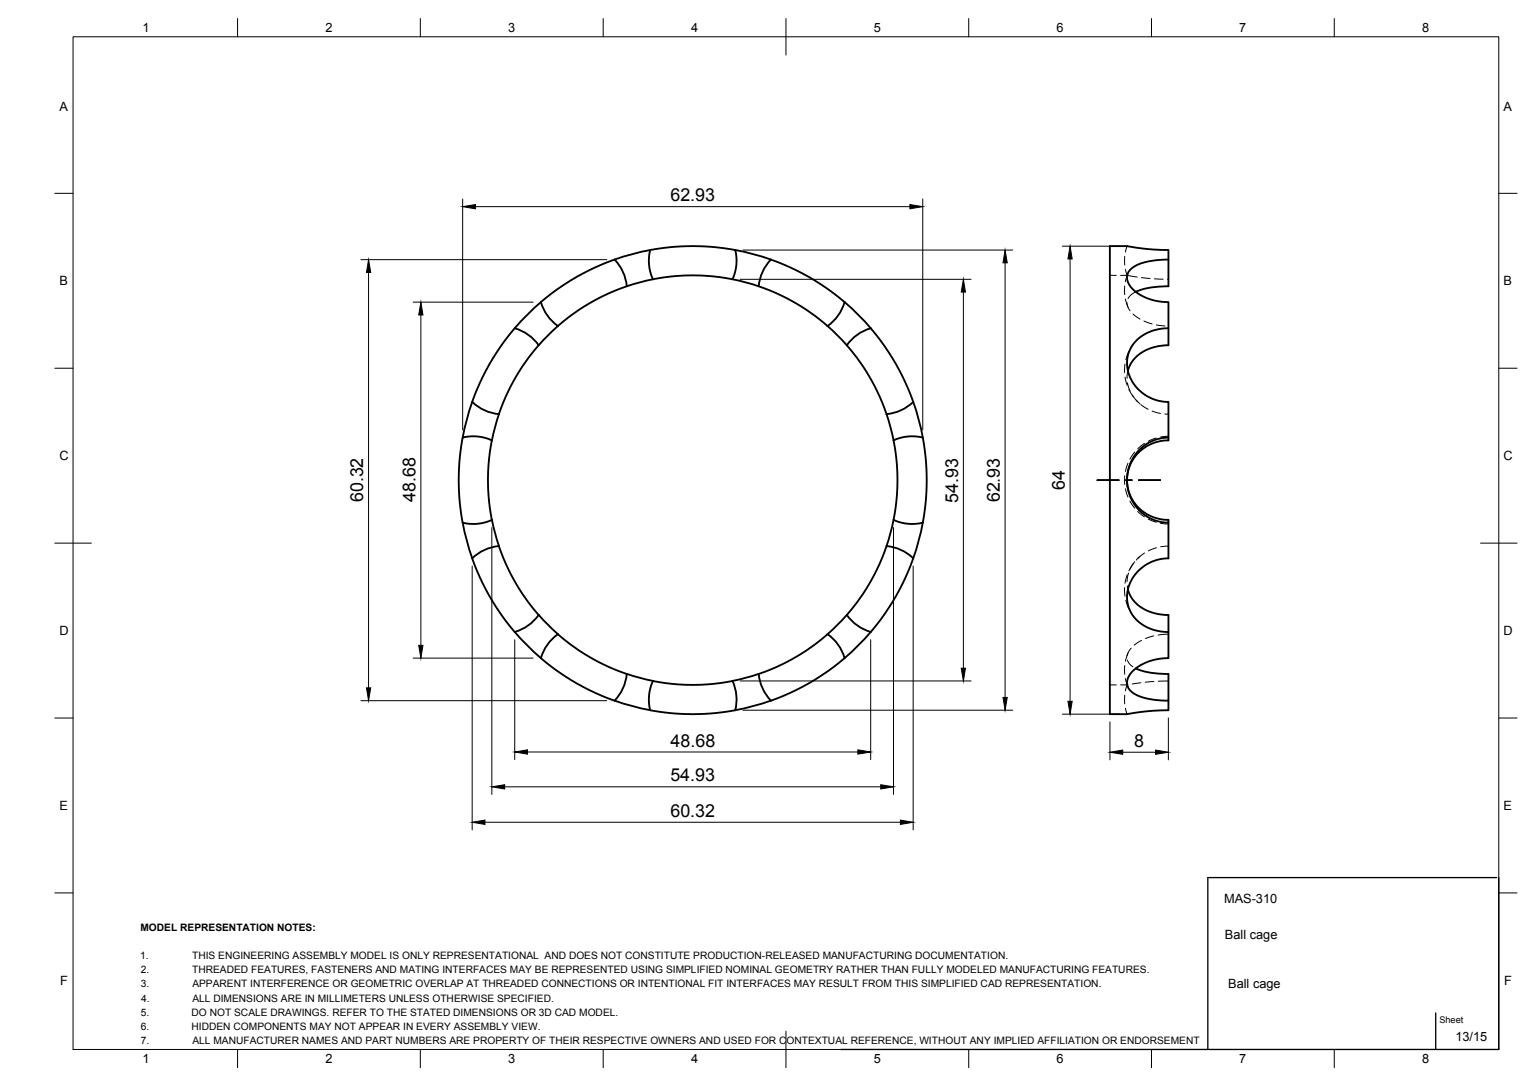
ISO-10303-21;
HEADER;
/* Generated by software containing ST-Developer
 * from STEP Tools, Inc. (www.steptools.com) 
 */

FILE_DESCRIPTION(
/* description */ ('Independent30mm screw-fed quill/spindle unit with16mm straight tool s
ocket, radial set screw, native reusable open ball bearings, retained 
inner/outer race stacks, keyed quill guide and M12x1.75 fine feed. Ext
ernal moving drive and tool not included. Ideal cage orbital links; in
dividual ball spin, force and preload not simulated. No drilling capac
ity, runout, speed, torque, load, life or machine safety rating.'),
/* implementation_level */ '2;1');

FILE_NAME(
/* name */ 'Ball cage.step',
/* time_stamp */ '2026-11-08T18:59:42-08:00',
/* author */ (''),
/* organization */ (''),
/* preprocessor_version */ 'ST-DEVELOPER v20.2',
/* originating_system */ 'Autodesk Translation Framework v15.17.0.0',
/* authorisation */ '');

FILE_SCHEMA (('AUTOMOTIVE_DESIGN { 1 0 10303 214 3 1 1 }'));
ENDSEC;

DATA;
#10=MECHANICAL_DESIGN_GEOMETRIC_PRESENTATION_REPRESENTATION('',(#1607),#63898);
#224=SPHERICAL_SURFACE('',#16652,6.);
#225=SPHERICAL_SURFACE('',#16673,6.);
#226=SPHERICAL_SURFACE('',#16679,6.);
#227=SPHERICAL_SURFACE('',#16686,6.);
#228=SPHERICAL_SURFACE('',#16692,6.);
#229=SPHERICAL_SURFACE('',#16698,6.);
#230=SPHERICAL_SURFACE('',#16704,6.);
#231=SPHERICAL_SURFACE('',#16710,6.);
#232=SPHERICAL_SURFACE('',#16717,6.);
#233=SPHERICAL_SURFACE('',#16723,6.);
#234=SPHERICAL_SURFACE('',#16729,6.);
#235=SPHERICAL_SURFACE('',#16735,6.);
#1448=B_SPLINE_CURVE_WITH_KNOTS('',3,(#60434,#60435,#60436,#60437,#60438,
#60439,#60440,#60441,#60442,#60443,#60444,#60445,#60446,#60447,#60448,#60449,
#60450,#60451,#60452,#60453,#60454,#60455,#60456,#60457,#60458,#60459),
 .UNSPECIFIED.,.F.,.F.,(4,2,2,2,2,2,2,2,2,2,2,2,4),(-1.71701449155744,-1.52195735713249,
-1.32690022270754,-1.23846982832783,-1.15003943394813,-1.00427333986342,
-0.858507245778717,-0.712741151694014,-0.56697505760931,-0.478544663229604,
-0.390114268849898,-0.195057134424949,0.),.UNSPECIFIED.);
#1449=B_SPLINE_CURVE_WITH_KNOTS('',3,(#60463,#60464,#60465,#60466,#60467,
#60468,#60469,#60470,#60471,#60472,#60473,#60474),.UNSPECIFIED.,.F.,.F.,
(4,2,2,2,2,4),(-0.73325034842368,-0.710785333485644,-0.57603622531241,-0.432027168984308,
-0.288018112656205,0.),.UNSPECIFIED.);
#1450=B_SPLINE_CURVE_WITH_KNOTS('',3,(#60478,#60479,#60480,#60481,#60482,
#60483,#60484,#60485,#60486,#60487,#60488,#60489,#60490,#60491),
 .UNSPECIFIED.,.F.,.F.,(4,2,2,2,2,2,4),(-1.69106888331775,-1.40305077066155,
-1.25904171433345,-1.11503265800535,-0.980283549832111,-0.845534441658878,
-0.73325034842368),.UNSPECIFIED.);
#1451=B_SPLINE_CURVE_WITH_KNOTS('',3,(#60499,#60500,#60501,#60502,#60503,
#60504,#60505,#60506,#60507,#60508,#60509,#60510),.UNSPECIFIED.,.F.,.F.,
(4,2,2,2,2,4),(-0.845534441658877,-0.710785333485644,-0.576036225312411,
-0.432027168984308,-0.288018112656205,0.),.UNSPECIFIED.);
#1452=B_SPLINE_CURVE_WITH_KNOTS('',3,(#60514,#60515,#60516,#60517,#60518,
#60519,#60520,#60521,#60522,#60523,#60524,#60525,#60526,#60527,#60528,#60529,
#60530,#60531,#60532,#60533,#60534,#60535),.UNSPECIFIED.,.F.,.F.,(4,2,2,
2,2,2,2,2,2,2,4),(-1.69106888331776,-1.40305077066155,-1.25904171433345,
-1.11503265800535,-0.980283549832111,-0.845534441658878,-0.710785333485644,
-0.57603622531241,-0.432027168984307,-0.288018112656205,0.),
 .UNSPECIFIED.);
#1453=B_SPLINE_CURVE_WITH_KNOTS('',3,(#60539,#60540,#60541,#60542,#60543,
#60544,#60545,#60546,#60547,#60548,#60549,#60550,#60551,#60552,#60553,#60554,
#60555,#60556,#60557,#60558,#60559,#60560),.UNSPECIFIED.,.F.,.F.,(4,2,2,
2,2,2,2,2,2,2,4),(-1.69106888331776,-1.40305077066155,-1.25904171433345,
-1.11503265800535,-0.980283549832111,-0.845534441658878,-0.710785333485644,
-0.57603622531241,-0.432027168984307,-0.288018112656205,0.),
 .UNSPECIFIED.);
#1454=B_SPLINE_CURVE_WITH_KNOTS('',3,(#60564,#60565,#60566,#60567,#60568,
#60569,#60570,#60571,#60572,#60573,#60574,#60575,#60576,#60577,#60578,#60579,
#60580,#60581,#60582,#60583,#60584,#60585),.UNSPECIFIED.,.F.,.F.,(4,2,2,
2,2,2,2,2,2,2,4),(-1.69106888331775,-1.40305077066155,-1.25904171433345,
-1.11503265800534,-0.980283549832111,-0.845534441658877,-0.710785333485644,
-0.57603622531241,-0.432027168984307,-0.288018112656205,0.),
 .UNSPECIFIED.);
#1455=B_SPLINE_CURVE_WITH_KNOTS('',3,(#60589,#60590,#60591,#60592,#60593,
#60594),.UNSPECIFIED.,.F.,.F.,(4,2,4),(-1.69106888331776,-1.40305077066155,
-1.27424252614337),.UNSPECIFIED.);
#1456=B_SPLINE_CURVE_WITH_KNOTS('',3,(#60596,#60597,#60598,#60599,#60600,
#60601,#60602,#60603,#60604,#60605,#60606,#60607,#60608,#60609,#60610,#60611,
#60612,#60613,#60614,#60615),.UNSPECIFIED.,.F.,.F.,(4,2,2,2,2,2,2,2,2,4),
(-1.27424252614337,-1.25904171433345,-1.11503265800534,-0.980283549832111,
-0.845534441658877,-0.710785333485643,-0.576036225312409,-0.432027168984307,
-0.288018112656205,0.),.UNSPECIFIED.);
#1457=B_SPLINE_CURVE_WITH_KNOTS('',3,(#60619,#60620,#60621,#60622,#60623,
#60624,#60625,#60626,#60627,#60628,#60629,#60630),.UNSPECIFIED.,.F.,.F.,
(4,2,2,2,2,4),(-1.69106888331776,-1.40305077066155,-1.25904171433345,-1.11503265800534,
-0.980283549832111,-0.957818534894075),.UNSPECIFIED.);
#1458=B_SPLINE_CURVE_WITH_KNOTS('',3,(#60632,#60633,#60634,#60635,#60636,
#60637,#60638,#60639,#60640,#60641,#60642,#60643,#60644,#60645),
 .UNSPECIFIED.,.F.,.F.,(4,2,2,2,2,2,4),(-0.957818534894075,-0.845534441658877,
-0.710785333485644,-0.57603622531241,-0.432027168984307,-0.288018112656205,
0.),.UNSPECIFIED.);
#1459=B_SPLINE_CURVE_WITH_KNOTS('',3,(#60649,#60650,#60651,#60652,#60653,
#60654,#60655,#60656,#60657,#60658,#60659,#60660),.UNSPECIFIED.,.F.,.F.,
(4,2,2,2,2,4),(-1.69106888331776,-1.40305077066155,-1.25904171433345,-1.11503265800535,
-0.980283549832111,-0.845534441658878),.UNSPECIFIED.);
#1460=B_SPLINE_CURVE_WITH_KNOTS('',3,(#60662,#60663,#60664,#60665,#60666,
#60667,#60668,#60669,#60670,#60671,#60672,#60673),.UNSPECIFIED.,.F.,.F.,
(4,2,2,2,2,4),(-0.845534441658878,-0.710785333485644,-0.57603622531241,
-0.432027168984308,-0.288018112656205,0.),.UNSPECIFIED.);
#1461=B_SPLINE_CURVE_WITH_KNOTS('',3,(#60678,#60679,#60680,#60681,#60682,
#60683,#60684,#60685,#60686,#60687,#60688,#60689,#60690,#60691,#60692,#60693,
#60694,#60695,#60696,#60697),.UNSPECIFIED.,.F.,.F.,(4,2,2,2,2,2,2,2,2,4),
(-1.69106888331775,-1.40305077066155,-1.25904171433345,-1.11503265800535,
-0.980283549832112,-0.845534441658878,-0.710785333485644,-0.57603622531241,
-0.432027168984308,-0.416826357174388),.UNSPECIFIED.);
#1462=B_SPLINE_CURVE_WITH_KNOTS('',3,(#60699,#60700,#60701,#60702,#60703,
#60704),.UNSPECIFIED.,.F.,.F.,(4,2,4),(-0.416826357174388,-0.288018112656205,
0.),.UNSPECIFIED.);
#1463=B_SPLINE_CURVE_WITH_KNOTS('',3,(#60708,#60709,#60710,#60711,#60712,
#60713,#60714,#60715,#60716,#60717,#60718,#60719,#60720,#60721,#60722,#60723,
#60724,#60725,#60726,#60727,#60728,#60729),.UNSPECIFIED.,.F.,.F.,(4,2,2,
2,2,2,2,2,2,2,4),(-1.69106888331776,-1.40305077066155,-1.25904171433345,
-1.11503265800535,-0.980283549832111,-0.845534441658878,-0.710785333485644,
-0.576036225312411,-0.432027168984308,-0.288018112656205,0.),
 .UNSPECIFIED.);
#1464=B_SPLINE_CURVE_WITH_KNOTS('',3,(#60733,#60734,#60735,#60736,#60737,
#60738,#60739,#60740,#60741,#60742,#60743,#60744,#60745,#60746,#60747,#60748,
#60749,#60750,#60751,#60752,#60753,#60754),.UNSPECIFIED.,.F.,.F.,(4,2,2,
2,2,2,2,2,2,2,4),(-1.69106888331776,-1.40305077066155,-1.25904171433345,
-1.11503265800535,-0.980283549832111,-0.845534441658878,-0.710785333485644,
-0.57603622531241,-0.432027168984308,-0.288018112656205,0.),
 .UNSPECIFIED.);
#1465=B_SPLINE_CURVE_WITH_KNOTS('',3,(#60758,#60759,#60760,#60761,#60762,
#60763,#60764,#60765,#60766,#60767,#60768,#60769,#60770,#60771,#60772,#60773,
#60774,#60775,#60776,#60777,#60778,#60779),.UNSPECIFIED.,.F.,.F.,(4,2,2,
2,2,2,2,2,2,2,4),(-1.69106888331776,-1.40305077066155,-1.25904171433345,
-1.11503265800535,-0.980283549832113,-0.845534441658879,-0.710785333485645,
-0.576036225312412,-0.432027168984308,-0.288018112656206,0.),
 .UNSPECIFIED.);
#1466=B_SPLINE_CURVE_WITH_KNOTS('',3,(#60782,#60783,#60784,#60785,#60786,
#60787,#60788,#60789,#60790,#60791,#60792,#60793),.UNSPECIFIED.,.F.,.F.,
(4,2,2,2,2,4),(-1.69106888331776,-1.40305077066155,-1.25904171433345,-1.11503265800535,
-0.980283549832112,-0.845534441658877),.UNSPECIFIED.);
#1467=B_SPLINE_CURVE_WITH_KNOTS('',3,(#60800,#60801,#60802,#60803,#60804,
#60805,#60806,#60807,#60808,#60809,#60810,#60811,#60812,#60813,#60814,#60815,
#60816,#60817,#60818,#60819,#60820,#60821,#60822,#60823,#60824,#60825),
 .UNSPECIFIED.,.F.,.F.,(4,2,2,2,2,2,2,2,2,2,2,2,4),(-1.71701449155743,-1.52195735713249,
-1.32690022270754,-1.23846982832783,-1.15003943394812,-1.00427333986342,
-0.858507245778717,-0.712741151694013,-0.56697505760931,-0.478544663229604,
-0.390114268849898,-0.195057134424949,0.),.UNSPECIFIED.);
#1468=B_SPLINE_CURVE_WITH_KNOTS('',3,(#60835,#60836,#60837,#60838,#60839,
#60840,#60841,#60842,#60843,#60844,#60845,#60846,#60847,#60848,#60849,#60850,
#60851,#60852,#60853,#60854,#60855,#60856,#60857,#60858,#60859,#60860),
 .UNSPECIFIED.,.F.,.F.,(4,2,2,2,2,2,2,2,2,2,2,2,4),(-1.71701449155744,-1.52195735713249,
-1.32690022270754,-1.23846982832783,-1.15003943394812,-1.00427333986342,
-0.858507245778718,-0.712741151694014,-0.56697505760931,-0.478544663229604,
-0.390114268849898,-0.195057134424949,0.),.UNSPECIFIED.);
#1469=B_SPLINE_CURVE_WITH_KNOTS('',3,(#60873,#60874,#60875,#60876,#60877,
#60878,#60879,#60880,#60881,#60882),.UNSPECIFIED.,.F.,.F.,(4,2,2,2,4),(-1.71701449155744,
-1.52195735713249,-1.32690022270754,-1.23846982832783,-1.17815521207059),
 .UNSPECIFIED.);
#1470=B_SPLINE_CURVE_WITH_KNOTS('',3,(#60884,#60885,#60886,#60887,#60888,
#60889,#60890,#60891,#60892,#60893,#60894,#60895,#60896,#60897,#60898,#60899,
#60900,#60901,#60902,#60903),.UNSPECIFIED.,.F.,.F.,(4,2,2,2,2,2,2,2,2,4),
(-1.17815521207059,-1.15003943394812,-1.00427333986342,-0.858507245778718,
-0.712741151694014,-0.56697505760931,-0.478544663229604,-0.390114268849898,
-0.195057134424949,0.),.UNSPECIFIED.);
#1471=B_SPLINE_CURVE_WITH_KNOTS('',3,(#60913,#60914,#60915,#60916,#60917,
#60918,#60919,#60920,#60921,#60922,#60923,#60924,#60925,#60926),
 .UNSPECIFIED.,.F.,.F.,(4,2,2,2,2,2,4),(-1.71701449155744,-1.52195735713249,
-1.32690022270754,-1.23846982832783,-1.15003943394813,-1.00427333986342,
-0.968278936736989),.UNSPECIFIED.);
#1472=B_SPLINE_CURVE_WITH_KNOTS('',3,(#60928,#60929,#60930,#60931,#60932,
#60933,#60934,#60935,#60936,#60937,#60938,#60939,#60940,#60941,#60942,#60943),
 .UNSPECIFIED.,.F.,.F.,(4,2,2,2,2,2,2,4),(-0.968278936736989,-0.858507245778719,
-0.712741151694015,-0.566975057609311,-0.478544663229605,-0.390114268849899,
-0.19505713442495,0.),.UNSPECIFIED.);
#1473=B_SPLINE_CURVE_WITH_KNOTS('',3,(#60953,#60954,#60955,#60956,#60957,
#60958,#60959,#60960,#60961,#60962,#60963,#60964,#60965,#60966),
 .UNSPECIFIED.,.F.,.F.,(4,2,2,2,2,2,4),(-1.71701449155743,-1.52195735713248,
-1.32690022270754,-1.23846982832783,-1.15003943394812,-1.00427333986342,
-0.858507245778716),.UNSPECIFIED.);
#1474=B_SPLINE_CURVE_WITH_KNOTS('',3,(#60968,#60969,#60970,#60971,#60972,
#60973,#60974,#60975,#60976,#60977,#60978,#60979,#60980,#60981),
 .UNSPECIFIED.,.F.,.F.,(4,2,2,2,2,2,4),(-0.858507245778716,-0.712741151694012,
-0.566975057609308,-0.478544663229602,-0.390114268849896,-0.195057134424948,
0.),.UNSPECIFIED.);
#1475=B_SPLINE_CURVE_WITH_KNOTS('',3,(#60991,#60992,#60993,#60994,#60995,
#60996,#60997,#60998,#60999,#61000,#61001,#61002,#61003,#61004,#61005,#61006),
 .UNSPECIFIED.,.F.,.F.,(4,2,2,2,2,2,2,4),(-1.71701449155744,-1.52195735713249,
-1.32690022270754,-1.23846982832783,-1.15003943394812,-1.00427333986342,
-0.858507245778716,-0.748735554820447),.UNSPECIFIED.);
#1476=B_SPLINE_CURVE_WITH_KNOTS('',3,(#61008,#61009,#61010,#61011,#61012,
#61013,#61014,#61015,#61016,#61017,#61018,#61019,#61020,#61021),
 .UNSPECIFIED.,.F.,.F.,(4,2,2,2,2,2,4),(-0.748735554820447,-0.712741151694013,
-0.56697505760931,-0.478544663229603,-0.390114268849895,-0.195057134424948,
0.),.UNSPECIFIED.);
#1477=B_SPLINE_CURVE_WITH_KNOTS('',3,(#61031,#61032,#61033,#61034,#61035,
#61036,#61037,#61038,#61039,#61040,#61041,#61042,#61043,#61044,#61045,#61046,
#61047,#61048,#61049,#61050),.UNSPECIFIED.,.F.,.F.,(4,2,2,2,2,2,2,2,2,4),
(-1.71701449155743,-1.52195735713249,-1.32690022270754,-1.23846982832783,
-1.15003943394812,-1.00427333986342,-0.858507245778717,-0.712741151694014,
-0.566975057609311,-0.538859279486847),.UNSPECIFIED.);
#1478=B_SPLINE_CURVE_WITH_KNOTS('',3,(#61052,#61053,#61054,#61055,#61056,
#61057,#61058,#61059,#61060,#61061),.UNSPECIFIED.,.F.,.F.,(4,2,2,2,4),(-0.538859279486847,
-0.478544663229605,-0.3901142688499,-0.19505713442495,0.),.UNSPECIFIED.);
#1479=B_SPLINE_CURVE_WITH_KNOTS('',3,(#61072,#61073,#61074,#61075,#61076,
#61077,#61078,#61079,#61080,#61081,#61082,#61083,#61084,#61085,#61086,#61087,
#61088,#61089,#61090,#61091,#61092,#61093,#61094,#61095,#61096,#61097),
 .UNSPECIFIED.,.F.,.F.,(4,2,2,2,2,2,2,2,2,2,2,2,4),(-1.71701449155743,-1.52195735713249,
-1.32690022270754,-1.23846982832783,-1.15003943394813,-1.00427333986342,
-0.858507245778717,-0.712741151694013,-0.56697505760931,-0.478544663229603,
-0.390114268849897,-0.195057134424949,0.),.UNSPECIFIED.);
#1480=B_SPLINE_CURVE_WITH_KNOTS('',3,(#61107,#61108,#61109,#61110,#61111,
#61112,#61113,#61114,#61115,#61116,#61117,#61118,#61119,#61120,#61121,#61122,
#61123,#61124,#61125,#61126,#61127,#61128,#61129,#61130,#61131,#61132),
 .UNSPECIFIED.,.F.,.F.,(4,2,2,2,2,2,2,2,2,2,2,2,4),(-1.71701449155743,-1.52195735713249,
-1.32690022270754,-1.23846982832783,-1.15003943394812,-1.00427333986342,
-0.858507245778718,-0.712741151694014,-0.56697505760931,-0.478544663229604,
-0.390114268849898,-0.195057134424949,0.),.UNSPECIFIED.);
#1481=B_SPLINE_CURVE_WITH_KNOTS('',3,(#61142,#61143,#61144,#61145,#61146,
#61147,#61148,#61149,#61150,#61151,#61152,#61153,#61154,#61155,#61156,#61157,
#61158,#61159,#61160,#61161,#61162,#61163,#61164,#61165,#61166,#61167),
 .UNSPECIFIED.,.F.,.F.,(4,2,2,2,2,2,2,2,2,2,2,2,4),(-1.71701449155744,-1.52195735713249,
-1.32690022270754,-1.23846982832783,-1.15003943394813,-1.00427333986342,
-0.858507245778718,-0.712741151694014,-0.56697505760931,-0.478544663229604,
-0.390114268849898,-0.195057134424949,0.),.UNSPECIFIED.);
#1482=B_SPLINE_CURVE_WITH_KNOTS('',3,(#61177,#61178,#61179,#61180,#61181,
#61182,#61183,#61184,#61185,#61186,#61187,#61188,#61189,#61190,#61191,#61192,
#61193,#61194,#61195,#61196,#61197,#61198,#61199,#61200,#61201,#61202),
 .UNSPECIFIED.,.F.,.F.,(4,2,2,2,2,2,2,2,2,2,2,2,4),(-1.71701449155743,-1.52195735713249,
-1.32690022270754,-1.23846982832783,-1.15003943394812,-1.00427333986342,
-0.858507245778717,-0.712741151694014,-0.56697505760931,-0.478544663229604,
-0.390114268849898,-0.195057134424949,0.),.UNSPECIFIED.);
#1571=SHAPE_REPRESENTATION_RELATIONSHIP('SRR','None',#64010,#1589);
#1589=ADVANCED_BREP_SHAPE_REPRESENTATION('',(#1625),#63895);
#1607=STYLED_ITEM('',(#64105),#1625);
#1625=MANIFOLD_SOLID_BREP('Body1',#15493);
#1710=FACE_BOUND('',#4365,.T.);
#2341=CYLINDRICAL_SURFACE('',#16656,28.);
#2342=CYLINDRICAL_SURFACE('',#16738,32.);
#2585=CIRCLE('',#16653,6.);
#2586=CIRCLE('',#16654,6.);
#2587=CIRCLE('',#16655,6.);
#2588=CIRCLE('',#16657,28.);
#2589=CIRCLE('',#16658,28.);
#2590=CIRCLE('',#16659,28.);
#2591=CIRCLE('',#16660,28.);
#2592=CIRCLE('',#16661,28.);
#2593=CIRCLE('',#16662,28.);
#2594=CIRCLE('',#16663,28.);
#2595=CIRCLE('',#16664,28.);
#2596=CIRCLE('',#16665,28.);
#2597=CIRCLE('',#16666,28.);
#2598=CIRCLE('',#16667,28.);
#2599=CIRCLE('',#16668,28.);
#2600=CIRCLE('',#16669,28.);
#2601=CIRCLE('',#16671,32.);
#2602=CIRCLE('',#16672,6.);
#2603=CIRCLE('',#16674,6.);
#2604=CIRCLE('',#16675,6.);
#2605=CIRCLE('',#16677,32.);
#2606=CIRCLE('',#16678,6.);
#2607=CIRCLE('',#16680,6.);
#2608=CIRCLE('',#16681,6.);
#2609=CIRCLE('',#16682,6.);
#2610=CIRCLE('',#16684,32.);
#2611=CIRCLE('',#16685,6.);
#2612=CIRCLE('',#16687,6.);
#2613=CIRCLE('',#16688,6.);
#2614=CIRCLE('',#16690,32.);
#2615=CIRCLE('',#16691,6.);
#2616=CIRCLE('',#16693,6.);
#2617=CIRCLE('',#16694,6.00000000000001);
#2618=CIRCLE('',#16696,32.);
#2619=CIRCLE('',#16697,6.);
#2620=CIRCLE('',#16699,6.);
#2621=CIRCLE('',#16700,6.);
#2622=CIRCLE('',#16702,32.);
#2623=CIRCLE('',#16703,6.);
#2624=CIRCLE('',#16705,6.);
#2625=CIRCLE('',#16706,6.);
#2626=CIRCLE('',#16708,32.);
#2627=CIRCLE('',#16709,6.);
#2628=CIRCLE('',#16711,6.);
#2629=CIRCLE('',#16712,6.);
#2630=CIRCLE('',#16714,32.);
#2631=CIRCLE('',#16715,6.);
#2632=CIRCLE('',#16716,6.);
#2633=CIRCLE('',#16718,6.);
#2634=CIRCLE('',#16719,6.);
#2635=CIRCLE('',#16721,32.);
#2636=CIRCLE('',#16722,6.);
#2637=CIRCLE('',#16724,6.);
#2638=CIRCLE('',#16725,6.);
#2639=CIRCLE('',#16727,32.);
#2640=CIRCLE('',#16728,6.);
#2641=CIRCLE('',#16730,6.);
#2642=CIRCLE('',#16731,6.);
#2643=CIRCLE('',#16733,32.);
#2644=CIRCLE('',#16734,6.);
#2645=CIRCLE('',#16736,6.);
#2646=CIRCLE('',#16737,6.);
#2647=CIRCLE('',#16739,32.);
#2648=CIRCLE('',#16740,32.);
#3419=FACE_OUTER_BOUND('',#4339,.T.);
#3420=FACE_OUTER_BOUND('',#4340,.T.);
#3421=FACE_OUTER_BOUND('',#4341,.T.);
#3422=FACE_OUTER_BOUND('',#4342,.T.);
#3423=FACE_OUTER_BOUND('',#4343,.T.);
#3424=FACE_OUTER_BOUND('',#4344,.T.);
#3425=FACE_OUTER_BOUND('',#4345,.T.);
#3426=FACE_OUTER_BOUND('',#4346,.T.);
#3427=FACE_OUTER_BOUND('',#4347,.T.);
#3428=FACE_OUTER_BOUND('',#4348,.T.);
#3429=FACE_OUTER_BOUND('',#4349,.T.);
#3430=FACE_OUTER_BOUND('',#4350,.T.);
#3431=FACE_OUTER_BOUND('',#4351,.T.);
#3432=FACE_OUTER_BOUND('',#4352,.T.);
#3433=FACE_OUTER_BOUND('',#4353,.T.);
#3434=FACE_OUTER_BOUND('',#4354,.T.);
#3435=FACE_OUTER_BOUND('',#4355,.T.);
#3436=FACE_OUTER_BOUND('',#4356,.T.);
#3437=FACE_OUTER_BOUND('',#4357,.T.);
#3438=FACE_OUTER_BOUND('',#4358,.T.);
#3439=FACE_OUTER_BOUND('',#4359,.T.);
#3440=FACE_OUTER_BOUND('',#4360,.T.);
#3441=FACE_OUTER_BOUND('',#4361,.T.);
#3442=FACE_OUTER_BOUND('',#4362,.T.);
#3443=FACE_OUTER_BOUND('',#4363,.T.);
#3444=FACE_OUTER_BOUND('',#4364,.T.);
#3445=FACE_OUTER_BOUND('',#4366,.T.);
#4339=EDGE_LOOP('',(#14032,#14033,#14034,#14035,#14036,#14037,#14038));
#4340=EDGE_LOOP('',(#14039,#14040,#14041,#14042,#14043,#14044,#14045,#14046,
#14047,#14048,#14049,#14050,#14051,#14052,#14053,#14054,#14055,#14056,#14057,
#14058,#14059,#14060,#14061,#14062,#14063,#14064,#14065,#14066,#14067,#14068,
#14069,#14070,#14071));
#4341=EDGE_LOOP('',(#14072,#14073,#14074,#14075));
#4342=EDGE_LOOP('',(#14076,#14077,#14078,#14079,#14080,#14081,#14082));
#4343=EDGE_LOOP('',(#14083,#14084,#14085,#14086));
#4344=EDGE_LOOP('',(#14087,#14088,#14089,#14090,#14091,#14092,#14093));
#4345=EDGE_LOOP('',(#14094,#14095,#14096,#14097,#14098));
#4346=EDGE_LOOP('',(#14099,#14100,#14101,#14102,#14103,#14104,#14105));
#4347=EDGE_LOOP('',(#14106,#14107,#14108,#14109));
#4348=EDGE_LOOP('',(#14110,#14111,#14112,#14113,#14114,#14115,#14116));
#4349=EDGE_LOOP('',(#14117,#14118,#14119,#14120));
#4350=EDGE_LOOP('',(#14121,#14122,#14123,#14124,#14125,#14126,#14127,#14128));
#4351=EDGE_LOOP('',(#14129,#14130,#14131,#14132));
#4352=EDGE_LOOP('',(#14133,#14134,#14135,#14136,#14137,#14138,#14139));
#4353=EDGE_LOOP('',(#14140,#14141,#14142,#14143));
#4354=EDGE_LOOP('',(#14144,#14145,#14146,#14147,#14148,#14149,#14150));
#4355=EDGE_LOOP('',(#14151,#14152,#14153,#14154,#14155));
#4356=EDGE_LOOP('',(#14156,#14157,#14158,#14159,#14160,#14161,#14162));
#4357=EDGE_LOOP('',(#14163,#14164,#14165,#14166));
#4358=EDGE_LOOP('',(#14167,#14168,#14169,#14170,#14171,#14172,#14173));
#4359=EDGE_LOOP('',(#14174,#14175,#14176,#14177));
#4360=EDGE_LOOP('',(#14178,#14179,#14180,#14181,#14182,#14183,#14184));
#4361=EDGE_LOOP('',(#14185,#14186,#14187,#14188));
#4362=EDGE_LOOP('',(#14189,#14190,#14191,#14192,#14193,#14194,#14195));
#4363=EDGE_LOOP('',(#14196,#14197,#14198,#14199,#14200,#14201,#14202,#14203,
#14204,#14205,#14206,#14207,#14208,#14209,#14210,#14211,#14212,#14213,#14214,
#14215,#14216,#14217,#14218,#14219,#14220,#14221,#14222,#14223,#14224,#14225,
#14226,#14227));
#4364=EDGE_LOOP('',(#14228));
#4365=EDGE_LOOP('',(#14229));
#4366=EDGE_LOOP('',(#14230,#14231,#14232,#14233));
#5130=LINE('',#60497,#5893);
#5131=LINE('',#61209,#5894);
#5893=VECTOR('',#19492,28.);
#5894=VECTOR('',#19657,32.);
#7344=VERTEX_POINT('',#60432);
#7345=VERTEX_POINT('',#60433);
#7346=VERTEX_POINT('',#60460);
#7347=VERTEX_POINT('',#60462);
#7348=VERTEX_POINT('',#60475);
#7349=VERTEX_POINT('',#60477);
#7350=VERTEX_POINT('',#60494);
#7351=VERTEX_POINT('',#60496);
#7352=VERTEX_POINT('',#60498);
#7353=VERTEX_POINT('',#60511);
#7354=VERTEX_POINT('',#60513);
#7355=VERTEX_POINT('',#60536);
#7356=VERTEX_POINT('',#60538);
#7357=VERTEX_POINT('',#60561);
#7358=VERTEX_POINT('',#60563);
#7359=VERTEX_POINT('',#60586);
#7360=VERTEX_POINT('',#60588);
#7361=VERTEX_POINT('',#60595);
#7362=VERTEX_POINT('',#60616);
#7363=VERTEX_POINT('',#60618);
#7364=VERTEX_POINT('',#60631);
#7365=VERTEX_POINT('',#60646);
#7366=VERTEX_POINT('',#60648);
#7367=VERTEX_POINT('',#60661);
#7368=VERTEX_POINT('',#60675);
#7369=VERTEX_POINT('',#60677);
#7370=VERTEX_POINT('',#60698);
#7371=VERTEX_POINT('',#60705);
#7372=VERTEX_POINT('',#60707);
#7373=VERTEX_POINT('',#60730);
#7374=VERTEX_POINT('',#60732);
#7375=VERTEX_POINT('',#60755);
#7376=VERTEX_POINT('',#60757);
#7377=VERTEX_POINT('',#60780);
#7378=VERTEX_POINT('',#60795);
#7379=VERTEX_POINT('',#60799);
#7380=VERTEX_POINT('',#60827);
#7381=VERTEX_POINT('',#60830);
#7382=VERTEX_POINT('',#60834);
#7383=VERTEX_POINT('',#60861);
#7384=VERTEX_POINT('',#60863);
#7385=VERTEX_POINT('',#60867);
#7386=VERTEX_POINT('',#60871);
#7387=VERTEX_POINT('',#60872);
#7388=VERTEX_POINT('',#60904);
#7389=VERTEX_POINT('',#60907);
#7390=VERTEX_POINT('',#60911);
#7391=VERTEX_POINT('',#60912);
#7392=VERTEX_POINT('',#60944);
#7393=VERTEX_POINT('',#60947);
#7394=VERTEX_POINT('',#60951);
#7395=VERTEX_POINT('',#60952);
#7396=VERTEX_POINT('',#60982);
#7397=VERTEX_POINT('',#60985);
#7398=VERTEX_POINT('',#60989);
#7399=VERTEX_POINT('',#60990);
#7400=VERTEX_POINT('',#61022);
#7401=VERTEX_POINT('',#61025);
#7402=VERTEX_POINT('',#61029);
#7403=VERTEX_POINT('',#61030);
#7404=VERTEX_POINT('',#61062);
#7405=VERTEX_POINT('',#61065);
#7406=VERTEX_POINT('',#61067);
#7407=VERTEX_POINT('',#61071);
#7408=VERTEX_POINT('',#61099);
#7409=VERTEX_POINT('',#61102);
#7410=VERTEX_POINT('',#61106);
#7411=VERTEX_POINT('',#61134);
#7412=VERTEX_POINT('',#61137);
#7413=VERTEX_POINT('',#61141);
#7414=VERTEX_POINT('',#61169);
#7415=VERTEX_POINT('',#61172);
#7416=VERTEX_POINT('',#61176);
#7417=VERTEX_POINT('',#61204);
#7418=VERTEX_POINT('',#61207);
#9605=EDGE_CURVE('',#7344,#7345,#1448,.T.);
#9606=EDGE_CURVE('',#7346,#7344,#2585,.T.);
#9607=EDGE_CURVE('',#7347,#7346,#1449,.T.);
#9608=EDGE_CURVE('',#7347,#7348,#2586,.T.);
#9609=EDGE_CURVE('',#7349,#7347,#1450,.T.);
#9610=EDGE_CURVE('',#7345,#7349,#2587,.T.);
#9611=EDGE_CURVE('',#7350,#7350,#2588,.T.);
#9612=EDGE_CURVE('',#7350,#7351,#5130,.T.);
#9613=EDGE_CURVE('',#7351,#7352,#1451,.T.);
#9614=EDGE_CURVE('',#7352,#7353,#2589,.T.);
#9615=EDGE_CURVE('',#7353,#7354,#1452,.T.);
#9616=EDGE_CURVE('',#7354,#7355,#2590,.T.);
#9617=EDGE_CURVE('',#7355,#7356,#1453,.T.);
#9618=EDGE_CURVE('',#7356,#7357,#2591,.T.);
#9619=EDGE_CURVE('',#7357,#7358,#1454,.T.);
#9620=EDGE_CURVE('',#7358,#7359,#2592,.T.);
#9621=EDGE_CURVE('',#7359,#7360,#1455,.T.);
#9622=EDGE_CURVE('',#7360,#7361,#1456,.T.);
#9623=EDGE_CURVE('',#7361,#7362,#2593,.T.);
#9624=EDGE_CURVE('',#7362,#7363,#1457,.T.);
#9625=EDGE_CURVE('',#7363,#7364,#1458,.T.);
#9626=EDGE_CURVE('',#7364,#7365,#2594,.T.);
#9627=EDGE_CURVE('',#7365,#7366,#1459,.T.);
#9628=EDGE_CURVE('',#7366,#7367,#1460,.T.);
#9629=EDGE_CURVE('',#7367,#7349,#2595,.T.);
#9630=EDGE_CURVE('',#7346,#7368,#2596,.T.);
#9631=EDGE_CURVE('',#7368,#7369,#1461,.T.);
#9632=EDGE_CURVE('',#7369,#7370,#1462,.T.);
#9633=EDGE_CURVE('',#7370,#7371,#2597,.T.);
#9634=EDGE_CURVE('',#7371,#7372,#1463,.T.);
#9635=EDGE_CURVE('',#7372,#7373,#2598,.T.);
#9636=EDGE_CURVE('',#7373,#7374,#1464,.T.);
#9637=EDGE_CURVE('',#7374,#7375,#2599,.T.);
#9638=EDGE_CURVE('',#7375,#7376,#1465,.T.);
#9639=EDGE_CURVE('',#7376,#7377,#2600,.T.);
#9640=EDGE_CURVE('',#7377,#7351,#1466,.T.);
#9641=EDGE_CURVE('',#7378,#7344,#2601,.T.);
#9642=EDGE_CURVE('',#7378,#7368,#2602,.T.);
#9643=EDGE_CURVE('',#7379,#7378,#1467,.T.);
#9644=EDGE_CURVE('',#7370,#7379,#2603,.T.);
#9645=EDGE_CURVE('',#7369,#7380,#2604,.T.);
#9646=EDGE_CURVE('',#7381,#7379,#2605,.T.);
#9647=EDGE_CURVE('',#7381,#7371,#2606,.T.);
#9648=EDGE_CURVE('',#7382,#7381,#1468,.T.);
#9649=EDGE_CURVE('',#7383,#7382,#2607,.T.);
#9650=EDGE_CURVE('',#7383,#7384,#2608,.T.);
#9651=EDGE_CURVE('',#7372,#7383,#2609,.T.);
#9652=EDGE_CURVE('',#7385,#7382,#2610,.T.);
#9653=EDGE_CURVE('',#7385,#7373,#2611,.T.);
#9654=EDGE_CURVE('',#7386,#7387,#1469,.T.);
#9655=EDGE_CURVE('',#7374,#7386,#2612,.T.);
#9656=EDGE_CURVE('',#7387,#7385,#1470,.T.);
#9657=EDGE_CURVE('',#7387,#7388,#2613,.T.);
#9658=EDGE_CURVE('',#7389,#7386,#2614,.T.);
#9659=EDGE_CURVE('',#7389,#7375,#2615,.T.);
#9660=EDGE_CURVE('',#7390,#7391,#1471,.T.);
#9661=EDGE_CURVE('',#7376,#7390,#2616,.T.);
#9662=EDGE_CURVE('',#7391,#7389,#1472,.T.);
#9663=EDGE_CURVE('',#7391,#7392,#2617,.T.);
#9664=EDGE_CURVE('',#7393,#7390,#2618,.T.);
#9665=EDGE_CURVE('',#7393,#7377,#2619,.T.);
#9666=EDGE_CURVE('',#7394,#7395,#1473,.T.);
#9667=EDGE_CURVE('',#7352,#7394,#2620,.T.);
#9668=EDGE_CURVE('',#7395,#7393,#1474,.T.);
#9669=EDGE_CURVE('',#7395,#7396,#2621,.T.);
#9670=EDGE_CURVE('',#7397,#7394,#2622,.T.);
#9671=EDGE_CURVE('',#7397,#7353,#2623,.T.);
#9672=EDGE_CURVE('',#7398,#7399,#1475,.T.);
#9673=EDGE_CURVE('',#7354,#7398,#2624,.T.);
#9674=EDGE_CURVE('',#7399,#7397,#1476,.T.);
#9675=EDGE_CURVE('',#7399,#7400,#2625,.T.);
#9676=EDGE_CURVE('',#7401,#7398,#2626,.T.);
#9677=EDGE_CURVE('',#7401,#7355,#2627,.T.);
#9678=EDGE_CURVE('',#7402,#7403,#1477,.T.);
#9679=EDGE_CURVE('',#7356,#7402,#2628,.T.);
#9680=EDGE_CURVE('',#7403,#7401,#1478,.T.);
#9681=EDGE_CURVE('',#7403,#7404,#2629,.T.);
#9682=EDGE_CURVE('',#7405,#7402,#2630,.T.);
#9683=EDGE_CURVE('',#7405,#7406,#2631,.T.);
#9684=EDGE_CURVE('',#7406,#7357,#2632,.T.);
#9685=EDGE_CURVE('',#7407,#7405,#1479,.T.);
#9686=EDGE_CURVE('',#7358,#7407,#2633,.T.);
#9687=EDGE_CURVE('',#7406,#7408,#2634,.T.);
#9688=EDGE_CURVE('',#7409,#7407,#2635,.T.);
#9689=EDGE_CURVE('',#7409,#7359,#2636,.T.);
#9690=EDGE_CURVE('',#7410,#7409,#1480,.T.);
#9691=EDGE_CURVE('',#7361,#7410,#2637,.T.);
#9692=EDGE_CURVE('',#7360,#7411,#2638,.T.);
#9693=EDGE_CURVE('',#7412,#7410,#2639,.T.);
#9694=EDGE_CURVE('',#7412,#7362,#2640,.T.);
#9695=EDGE_CURVE('',#7413,#7412,#1481,.T.);
#9696=EDGE_CURVE('',#7364,#7413,#2641,.T.);
#9697=EDGE_CURVE('',#7363,#7414,#2642,.T.);
#9698=EDGE_CURVE('',#7415,#7413,#2643,.T.);
#9699=EDGE_CURVE('',#7415,#7365,#2644,.T.);
#9700=EDGE_CURVE('',#7416,#7415,#1482,.T.);
#9701=EDGE_CURVE('',#7367,#7416,#2645,.T.);
#9702=EDGE_CURVE('',#7366,#7417,#2646,.T.);
#9703=EDGE_CURVE('',#7418,#7418,#2647,.T.);
#9704=EDGE_CURVE('',#7418,#7395,#5131,.T.);
#9705=EDGE_CURVE('',#7345,#7416,#2648,.T.);
#14032=ORIENTED_EDGE('',*,*,#9605,.F.);
#14033=ORIENTED_EDGE('',*,*,#9606,.F.);
#14034=ORIENTED_EDGE('',*,*,#9607,.F.);
#14035=ORIENTED_EDGE('',*,*,#9608,.T.);
#14036=ORIENTED_EDGE('',*,*,#9608,.F.);
#14037=ORIENTED_EDGE('',*,*,#9609,.F.);
#14038=ORIENTED_EDGE('',*,*,#9610,.F.);
#14039=ORIENTED_EDGE('',*,*,#9611,.F.);
#14040=ORIENTED_EDGE('',*,*,#9612,.T.);
#14041=ORIENTED_EDGE('',*,*,#9613,.T.);
#14042=ORIENTED_EDGE('',*,*,#9614,.T.);
#14043=ORIENTED_EDGE('',*,*,#9615,.T.);
#14044=ORIENTED_EDGE('',*,*,#9616,.T.);
#14045=ORIENTED_EDGE('',*,*,#9617,.T.);
#14046=ORIENTED_EDGE('',*,*,#9618,.T.);
#14047=ORIENTED_EDGE('',*,*,#9619,.T.);
#14048=ORIENTED_EDGE('',*,*,#9620,.T.);
#14049=ORIENTED_EDGE('',*,*,#9621,.T.);
#14050=ORIENTED_EDGE('',*,*,#9622,.T.);
#14051=ORIENTED_EDGE('',*,*,#9623,.T.);
#14052=ORIENTED_EDGE('',*,*,#9624,.T.);
#14053=ORIENTED_EDGE('',*,*,#9625,.T.);
#14054=ORIENTED_EDGE('',*,*,#9626,.T.);
#14055=ORIENTED_EDGE('',*,*,#9627,.T.);
#14056=ORIENTED_EDGE('',*,*,#9628,.T.);
#14057=ORIENTED_EDGE('',*,*,#9629,.T.);
#14058=ORIENTED_EDGE('',*,*,#9609,.T.);
#14059=ORIENTED_EDGE('',*,*,#9607,.T.);
#14060=ORIENTED_EDGE('',*,*,#9630,.T.);
#14061=ORIENTED_EDGE('',*,*,#9631,.T.);
#14062=ORIENTED_EDGE('',*,*,#9632,.T.);
#14063=ORIENTED_EDGE('',*,*,#9633,.T.);
#14064=ORIENTED_EDGE('',*,*,#9634,.T.);
#14065=ORIENTED_EDGE('',*,*,#9635,.T.);
#14066=ORIENTED_EDGE('',*,*,#9636,.T.);
#14067=ORIENTED_EDGE('',*,*,#9637,.T.);
#14068=ORIENTED_EDGE('',*,*,#9638,.T.);
#14069=ORIENTED_EDGE('',*,*,#9639,.T.);
#14070=ORIENTED_EDGE('',*,*,#9640,.T.);
#14071=ORIENTED_EDGE('',*,*,#9612,.F.);
#14072=ORIENTED_EDGE('',*,*,#9606,.T.);
#14073=ORIENTED_EDGE('',*,*,#9641,.F.);
#14074=ORIENTED_EDGE('',*,*,#9642,.T.);
#14075=ORIENTED_EDGE('',*,*,#9630,.F.);
#14076=ORIENTED_EDGE('',*,*,#9643,.F.);
#14077=ORIENTED_EDGE('',*,*,#9644,.F.);
#14078=ORIENTED_EDGE('',*,*,#9632,.F.);
#14079=ORIENTED_EDGE('',*,*,#9645,.T.);
#14080=ORIENTED_EDGE('',*,*,#9645,.F.);
#14081=ORIENTED_EDGE('',*,*,#9631,.F.);
#14082=ORIENTED_EDGE('',*,*,#9642,.F.);
#14083=ORIENTED_EDGE('',*,*,#9644,.T.);
#14084=ORIENTED_EDGE('',*,*,#9646,.F.);
#14085=ORIENTED_EDGE('',*,*,#9647,.T.);
#14086=ORIENTED_EDGE('',*,*,#9633,.F.);
#14087=ORIENTED_EDGE('',*,*,#9648,.F.);
#14088=ORIENTED_EDGE('',*,*,#9649,.F.);
#14089=ORIENTED_EDGE('',*,*,#9650,.T.);
#14090=ORIENTED_EDGE('',*,*,#9650,.F.);
#14091=ORIENTED_EDGE('',*,*,#9651,.F.);
#14092=ORIENTED_EDGE('',*,*,#9634,.F.);
#14093=ORIENTED_EDGE('',*,*,#9647,.F.);
#14094=ORIENTED_EDGE('',*,*,#9651,.T.);
#14095=ORIENTED_EDGE('',*,*,#9649,.T.);
#14096=ORIENTED_EDGE('',*,*,#9652,.F.);
#14097=ORIENTED_EDGE('',*,*,#9653,.T.);
#14098=ORIENTED_EDGE('',*,*,#9635,.F.);
#14099=ORIENTED_EDGE('',*,*,#9654,.F.);
#14100=ORIENTED_EDGE('',*,*,#9655,.F.);
#14101=ORIENTED_EDGE('',*,*,#9636,.F.);
#14102=ORIENTED_EDGE('',*,*,#9653,.F.);
#14103=ORIENTED_EDGE('',*,*,#9656,.F.);
#14104=ORIENTED_EDGE('',*,*,#9657,.T.);
#14105=ORIENTED_EDGE('',*,*,#9657,.F.);
#14106=ORIENTED_EDGE('',*,*,#9655,.T.);
#14107=ORIENTED_EDGE('',*,*,#9658,.F.);
#14108=ORIENTED_EDGE('',*,*,#9659,.T.);
#14109=ORIENTED_EDGE('',*,*,#9637,.F.);
#14110=ORIENTED_EDGE('',*,*,#9660,.F.);
#14111=ORIENTED_EDGE('',*,*,#9661,.F.);
#14112=ORIENTED_EDGE('',*,*,#9638,.F.);
#14113=ORIENTED_EDGE('',*,*,#9659,.F.);
#14114=ORIENTED_EDGE('',*,*,#9662,.F.);
#14115=ORIENTED_EDGE('',*,*,#9663,.T.);
#14116=ORIENTED_EDGE('',*,*,#9663,.F.);
#14117=ORIENTED_EDGE('',*,*,#9661,.T.);
#14118=ORIENTED_EDGE('',*,*,#9664,.F.);
#14119=ORIENTED_EDGE('',*,*,#9665,.T.);
#14120=ORIENTED_EDGE('',*,*,#9639,.F.);
#14121=ORIENTED_EDGE('',*,*,#9666,.F.);
#14122=ORIENTED_EDGE('',*,*,#9667,.F.);
#14123=ORIENTED_EDGE('',*,*,#9613,.F.);
#14124=ORIENTED_EDGE('',*,*,#9640,.F.);
#14125=ORIENTED_EDGE('',*,*,#9665,.F.);
#14126=ORIENTED_EDGE('',*,*,#9668,.F.);
#14127=ORIENTED_EDGE('',*,*,#9669,.T.);
#14128=ORIENTED_EDGE('',*,*,#9669,.F.);
#14129=ORIENTED_EDGE('',*,*,#9667,.T.);
#14130=ORIENTED_EDGE('',*,*,#9670,.F.);
#14131=ORIENTED_EDGE('',*,*,#9671,.T.);
#14132=ORIENTED_EDGE('',*,*,#9614,.F.);
#14133=ORIENTED_EDGE('',*,*,#9672,.F.);
#14134=ORIENTED_EDGE('',*,*,#9673,.F.);
#14135=ORIENTED_EDGE('',*,*,#9615,.F.);
#14136=ORIENTED_EDGE('',*,*,#9671,.F.);
#14137=ORIENTED_EDGE('',*,*,#9674,.F.);
#14138=ORIENTED_EDGE('',*,*,#9675,.T.);
#14139=ORIENTED_EDGE('',*,*,#9675,.F.);
#14140=ORIENTED_EDGE('',*,*,#9673,.T.);
#14141=ORIENTED_EDGE('',*,*,#9676,.F.);
#14142=ORIENTED_EDGE('',*,*,#9677,.T.);
#14143=ORIENTED_EDGE('',*,*,#9616,.F.);
#14144=ORIENTED_EDGE('',*,*,#9678,.F.);
#14145=ORIENTED_EDGE('',*,*,#9679,.F.);
#14146=ORIENTED_EDGE('',*,*,#9617,.F.);
#14147=ORIENTED_EDGE('',*,*,#9677,.F.);
#14148=ORIENTED_EDGE('',*,*,#9680,.F.);
#14149=ORIENTED_EDGE('',*,*,#9681,.T.);
#14150=ORIENTED_EDGE('',*,*,#9681,.F.);
#14151=ORIENTED_EDGE('',*,*,#9679,.T.);
#14152=ORIENTED_EDGE('',*,*,#9682,.F.);
#14153=ORIENTED_EDGE('',*,*,#9683,.T.);
#14154=ORIENTED_EDGE('',*,*,#9684,.T.);
#14155=ORIENTED_EDGE('',*,*,#9618,.F.);
#14156=ORIENTED_EDGE('',*,*,#9685,.F.);
#14157=ORIENTED_EDGE('',*,*,#9686,.F.);
#14158=ORIENTED_EDGE('',*,*,#9619,.F.);
#14159=ORIENTED_EDGE('',*,*,#9684,.F.);
#14160=ORIENTED_EDGE('',*,*,#9687,.T.);
#14161=ORIENTED_EDGE('',*,*,#9687,.F.);
#14162=ORIENTED_EDGE('',*,*,#9683,.F.);
#14163=ORIENTED_EDGE('',*,*,#9686,.T.);
#14164=ORIENTED_EDGE('',*,*,#9688,.F.);
#14165=ORIENTED_EDGE('',*,*,#9689,.T.);
#14166=ORIENTED_EDGE('',*,*,#9620,.F.);
#14167=ORIENTED_EDGE('',*,*,#9690,.F.);
#14168=ORIENTED_EDGE('',*,*,#9691,.F.);
#14169=ORIENTED_EDGE('',*,*,#9622,.F.);
#14170=ORIENTED_EDGE('',*,*,#9692,.T.);
#14171=ORIENTED_EDGE('',*,*,#9692,.F.);
#14172=ORIENTED_EDGE('',*,*,#9621,.F.);
#14173=ORIENTED_EDGE('',*,*,#9689,.F.);
#14174=ORIENTED_EDGE('',*,*,#9691,.T.);
#14175=ORIENTED_EDGE('',*,*,#9693,.F.);
#14176=ORIENTED_EDGE('',*,*,#9694,.T.);
#14177=ORIENTED_EDGE('',*,*,#9623,.F.);
#14178=ORIENTED_EDGE('',*,*,#9695,.F.);
#14179=ORIENTED_EDGE('',*,*,#9696,.F.);
#14180=ORIENTED_EDGE('',*,*,#9625,.F.);
#14181=ORIENTED_EDGE('',*,*,#9697,.T.);
#14182=ORIENTED_EDGE('',*,*,#9697,.F.);
#14183=ORIENTED_EDGE('',*,*,#9624,.F.);
#14184=ORIENTED_EDGE('',*,*,#9694,.F.);
#14185=ORIENTED_EDGE('',*,*,#9696,.T.);
#14186=ORIENTED_EDGE('',*,*,#9698,.F.);
#14187=ORIENTED_EDGE('',*,*,#9699,.T.);
#14188=ORIENTED_EDGE('',*,*,#9626,.F.);
#14189=ORIENTED_EDGE('',*,*,#9700,.F.);
#14190=ORIENTED_EDGE('',*,*,#9701,.F.);
#14191=ORIENTED_EDGE('',*,*,#9628,.F.);
#14192=ORIENTED_EDGE('',*,*,#9702,.T.);
#14193=ORIENTED_EDGE('',*,*,#9702,.F.);
#14194=ORIENTED_EDGE('',*,*,#9627,.F.);
#14195=ORIENTED_EDGE('',*,*,#9699,.F.);
#14196=ORIENTED_EDGE('',*,*,#9703,.F.);
#14197=ORIENTED_EDGE('',*,*,#9704,.T.);
#14198=ORIENTED_EDGE('',*,*,#9668,.T.);
#14199=ORIENTED_EDGE('',*,*,#9664,.T.);
#14200=ORIENTED_EDGE('',*,*,#9660,.T.);
#14201=ORIENTED_EDGE('',*,*,#9662,.T.);
#14202=ORIENTED_EDGE('',*,*,#9658,.T.);
#14203=ORIENTED_EDGE('',*,*,#9654,.T.);
#14204=ORIENTED_EDGE('',*,*,#9656,.T.);
#14205=ORIENTED_EDGE('',*,*,#9652,.T.);
#14206=ORIENTED_EDGE('',*,*,#9648,.T.);
#14207=ORIENTED_EDGE('',*,*,#9646,.T.);
#14208=ORIENTED_EDGE('',*,*,#9643,.T.);
#14209=ORIENTED_EDGE('',*,*,#9641,.T.);
#14210=ORIENTED_EDGE('',*,*,#9605,.T.);
#14211=ORIENTED_EDGE('',*,*,#9705,.T.);
#14212=ORIENTED_EDGE('',*,*,#9700,.T.);
#14213=ORIENTED_EDGE('',*,*,#9698,.T.);
#14214=ORIENTED_EDGE('',*,*,#9695,.T.);
#14215=ORIENTED_EDGE('',*,*,#9693,.T.);
#14216=ORIENTED_EDGE('',*,*,#9690,.T.);
#14217=ORIENTED_EDGE('',*,*,#9688,.T.);
#14218=ORIENTED_EDGE('',*,*,#9685,.T.);
#14219=ORIENTED_EDGE('',*,*,#9682,.T.);
#14220=ORIENTED_EDGE('',*,*,#9678,.T.);
#14221=ORIENTED_EDGE('',*,*,#9680,.T.);
#14222=ORIENTED_EDGE('',*,*,#9676,.T.);
#14223=ORIENTED_EDGE('',*,*,#9672,.T.);
#14224=ORIENTED_EDGE('',*,*,#9674,.T.);
#14225=ORIENTED_EDGE('',*,*,#9670,.T.);
#14226=ORIENTED_EDGE('',*,*,#9666,.T.);
#14227=ORIENTED_EDGE('',*,*,#9704,.F.);
#14228=ORIENTED_EDGE('',*,*,#9703,.T.);
#14229=ORIENTED_EDGE('',*,*,#9611,.T.);
#14230=ORIENTED_EDGE('',*,*,#9610,.T.);
#14231=ORIENTED_EDGE('',*,*,#9629,.F.);
#14232=ORIENTED_EDGE('',*,*,#9701,.T.);
#14233=ORIENTED_EDGE('',*,*,#9705,.F.);
#14615=PLANE('',#16670);
#14616=PLANE('',#16676);
#14617=PLANE('',#16683);
#14618=PLANE('',#16689);
#14619=PLANE('',#16695);
#14620=PLANE('',#16701);
#14621=PLANE('',#16707);
#14622=PLANE('',#16713);
#14623=PLANE('',#16720);
#14624=PLANE('',#16726);
#14625=PLANE('',#16732);
#14626=PLANE('',#16741);
#14627=PLANE('',#16742);
#15399=ADVANCED_FACE('',(#3419),#224,.F.);
#15400=ADVANCED_FACE('',(#3420),#2341,.F.);
#15401=ADVANCED_FACE('',(#3421),#14615,.F.);
#15402=ADVANCED_FACE('',(#3422),#225,.F.);
#15403=ADVANCED_FACE('',(#3423),#14616,.F.);
#15404=ADVANCED_FACE('',(#3424),#226,.F.);
#15405=ADVANCED_FACE('',(#3425),#14617,.F.);
#15406=ADVANCED_FACE('',(#3426),#227,.F.);
#15407=ADVANCED_FACE('',(#3427),#14618,.F.);
#15408=ADVANCED_FACE('',(#3428),#228,.F.);
#15409=ADVANCED_FACE('',(#3429),#14619,.F.);
#15410=ADVANCED_FACE('',(#3430),#229,.F.);
#15411=ADVANCED_FACE('',(#3431),#14620,.F.);
#15412=ADVANCED_FACE('',(#3432),#230,.F.);
#15413=ADVANCED_FACE('',(#3433),#14621,.F.);
#15414=ADVANCED_FACE('',(#3434),#231,.F.);
#15415=ADVANCED_FACE('',(#3435),#14622,.F.);
#15416=ADVANCED_FACE('',(#3436),#232,.F.);
#15417=ADVANCED_FACE('',(#3437),#14623,.F.);
#15418=ADVANCED_FACE('',(#3438),#233,.F.);
#15419=ADVANCED_FACE('',(#3439),#14624,.F.);
#15420=ADVANCED_FACE('',(#3440),#234,.F.);
#15421=ADVANCED_FACE('',(#3441),#14625,.F.);
#15422=ADVANCED_FACE('',(#3442),#235,.F.);
#15423=ADVANCED_FACE('',(#3443),#2342,.T.);
#15424=ADVANCED_FACE('',(#3444,#1710),#14626,.T.);
#15425=ADVANCED_FACE('',(#3445),#14627,.F.);
#15493=CLOSED_SHELL('',(#15399,#15400,#15401,#15402,#15403,#15404,#15405,
#15406,#15407,#15408,#15409,#15410,#15411,#15412,#15413,#15414,#15415,#15416,
#15417,#15418,#15419,#15420,#15421,#15422,#15423,#15424,#15425));
#16651=AXIS2_PLACEMENT_3D('',#60430,#19478,#19479);
#16652=AXIS2_PLACEMENT_3D('',#60431,#19480,#19481);
#16653=AXIS2_PLACEMENT_3D('',#60461,#19482,#19483);
#16654=AXIS2_PLACEMENT_3D('',#60476,#19484,#19485);
#16655=AXIS2_PLACEMENT_3D('',#60492,#19486,#19487);
#16656=AXIS2_PLACEMENT_3D('',#60493,#19488,#19489);
#16657=AXIS2_PLACEMENT_3D('',#60495,#19490,#19491);
#16658=AXIS2_PLACEMENT_3D('',#60512,#19493,#19494);
#16659=AXIS2_PLACEMENT_3D('',#60537,#19495,#19496);
#16660=AXIS2_PLACEMENT_3D('',#60562,#19497,#19498);
#16661=AXIS2_PLACEMENT_3D('',#60587,#19499,#19500);
#16662=AXIS2_PLACEMENT_3D('',#60617,#19501,#19502);
#16663=AXIS2_PLACEMENT_3D('',#60647,#19503,#19504);
#16664=AXIS2_PLACEMENT_3D('',#60674,#19505,#19506);
#16665=AXIS2_PLACEMENT_3D('',#60676,#19507,#19508);
#16666=AXIS2_PLACEMENT_3D('',#60706,#19509,#19510);
#16667=AXIS2_PLACEMENT_3D('',#60731,#19511,#19512);
#16668=AXIS2_PLACEMENT_3D('',#60756,#19513,#19514);
#16669=AXIS2_PLACEMENT_3D('',#60781,#19515,#19516);
#16670=AXIS2_PLACEMENT_3D('',#60794,#19517,#19518);
#16671=AXIS2_PLACEMENT_3D('',#60796,#19519,#19520);
#16672=AXIS2_PLACEMENT_3D('',#60797,#19521,#19522);
#16673=AXIS2_PLACEMENT_3D('',#60798,#19523,#19524);
#16674=AXIS2_PLACEMENT_3D('',#60826,#19525,#19526);
#16675=AXIS2_PLACEMENT_3D('',#60828,#19527,#19528);
#16676=AXIS2_PLACEMENT_3D('',#60829,#19529,#19530);
#16677=AXIS2_PLACEMENT_3D('',#60831,#19531,#19532);
#16678=AXIS2_PLACEMENT_3D('',#60832,#19533,#19534);
#16679=AXIS2_PLACEMENT_3D('',#60833,#19535,#19536);
#16680=AXIS2_PLACEMENT_3D('',#60862,#19537,#19538);
#16681=AXIS2_PLACEMENT_3D('',#60864,#19539,#19540);
#16682=AXIS2_PLACEMENT_3D('',#60865,#19541,#19542);
#16683=AXIS2_PLACEMENT_3D('',#60866,#19543,#19544);
#16684=AXIS2_PLACEMENT_3D('',#60868,#19545,#19546);
#16685=AXIS2_PLACEMENT_3D('',#60869,#19547,#19548);
#16686=AXIS2_PLACEMENT_3D('',#60870,#19549,#19550);
#16687=AXIS2_PLACEMENT_3D('',#60883,#19551,#19552);
#16688=AXIS2_PLACEMENT_3D('',#60905,#19553,#19554);
#16689=AXIS2_PLACEMENT_3D('',#60906,#19555,#19556);
#16690=AXIS2_PLACEMENT_3D('',#60908,#19557,#19558);
#16691=AXIS2_PLACEMENT_3D('',#60909,#19559,#19560);
#16692=AXIS2_PLACEMENT_3D('',#60910,#19561,#19562);
#16693=AXIS2_PLACEMENT_3D('',#60927,#19563,#19564);
#16694=AXIS2_PLACEMENT_3D('',#60945,#19565,#19566);
#16695=AXIS2_PLACEMENT_3D('',#60946,#19567,#19568);
#16696=AXIS2_PLACEMENT_3D('',#60948,#19569,#19570);
#16697=AXIS2_PLACEMENT_3D('',#60949,#19571,#19572);
#16698=AXIS2_PLACEMENT_3D('',#60950,#19573,#19574);
#16699=AXIS2_PLACEMENT_3D('',#60967,#19575,#19576);
#16700=AXIS2_PLACEMENT_3D('',#60983,#19577,#19578);
#16701=AXIS2_PLACEMENT_3D('',#60984,#19579,#19580);
#16702=AXIS2_PLACEMENT_3D('',#60986,#19581,#19582);
#16703=AXIS2_PLACEMENT_3D('',#60987,#19583,#19584);
#16704=AXIS2_PLACEMENT_3D('',#60988,#19585,#19586);
#16705=AXIS2_PLACEMENT_3D('',#61007,#19587,#19588);
#16706=AXIS2_PLACEMENT_3D('',#61023,#19589,#19590);
#16707=AXIS2_PLACEMENT_3D('',#61024,#19591,#19592);
#16708=AXIS2_PLACEMENT_3D('',#61026,#19593,#19594);
#16709=AXIS2_PLACEMENT_3D('',#61027,#19595,#19596);
#16710=AXIS2_PLACEMENT_3D('',#61028,#19597,#19598);
#16711=AXIS2_PLACEMENT_3D('',#61051,#19599,#19600);
#16712=AXIS2_PLACEMENT_3D('',#61063,#19601,#19602);
#16713=AXIS2_PLACEMENT_3D('',#61064,#19603,#19604);
#16714=AXIS2_PLACEMENT_3D('',#61066,#19605,#19606);
#16715=AXIS2_PLACEMENT_3D('',#61068,#19607,#19608);
#16716=AXIS2_PLACEMENT_3D('',#61069,#19609,#19610);
#16717=AXIS2_PLACEMENT_3D('',#61070,#19611,#19612);
#16718=AXIS2_PLACEMENT_3D('',#61098,#19613,#19614);
#16719=AXIS2_PLACEMENT_3D('',#61100,#19615,#19616);
#16720=AXIS2_PLACEMENT_3D('',#61101,#19617,#19618);
#16721=AXIS2_PLACEMENT_3D('',#61103,#19619,#19620);
#16722=AXIS2_PLACEMENT_3D('',#61104,#19621,#19622);
#16723=AXIS2_PLACEMENT_3D('',#61105,#19623,#19624);
#16724=AXIS2_PLACEMENT_3D('',#61133,#19625,#19626);
#16725=AXIS2_PLACEMENT_3D('',#61135,#19627,#19628);
#16726=AXIS2_PLACEMENT_3D('',#61136,#19629,#19630);
#16727=AXIS2_PLACEMENT_3D('',#61138,#19631,#19632);
#16728=AXIS2_PLACEMENT_3D('',#61139,#19633,#19634);
#16729=AXIS2_PLACEMENT_3D('',#61140,#19635,#19636);
#16730=AXIS2_PLACEMENT_3D('',#61168,#19637,#19638);
#16731=AXIS2_PLACEMENT_3D('',#61170,#19639,#19640);
#16732=AXIS2_PLACEMENT_3D('',#61171,#19641,#19642);
#16733=AXIS2_PLACEMENT_3D('',#61173,#19643,#19644);
#16734=AXIS2_PLACEMENT_3D('',#61174,#19645,#19646);
#16735=AXIS2_PLACEMENT_3D('',#61175,#19647,#19648);
#16736=AXIS2_PLACEMENT_3D('',#61203,#19649,#19650);
#16737=AXIS2_PLACEMENT_3D('',#61205,#19651,#19652);
#16738=AXIS2_PLACEMENT_3D('',#61206,#19653,#19654);
#16739=AXIS2_PLACEMENT_3D('',#61208,#19655,#19656);
#16740=AXIS2_PLACEMENT_3D('',#61210,#19658,#19659);
#16741=AXIS2_PLACEMENT_3D('',#61211,#19660,#19661);
#16742=AXIS2_PLACEMENT_3D('',#61212,#19662,#19663);
#19478=DIRECTION('axis',(0.,0.,1.));
#19479=DIRECTION('refdir',(1.,0.,0.));
#19480=DIRECTION('center_axis',(0.,0.,1.));
#19481=DIRECTION('ref_axis',(1.,0.,0.));
#19482=DIRECTION('center_axis',(0.,0.,1.));
#19483=DIRECTION('ref_axis',(0.,-1.,0.));
#19484=DIRECTION('center_axis',(0.,1.,0.));
#19485=DIRECTION('ref_axis',(-1.,0.,0.));
#19486=DIRECTION('center_axis',(0.,0.,1.));
#19487=DIRECTION('ref_axis',(0.,-1.,0.));
#19488=DIRECTION('center_axis',(0.,0.,1.));
#19489=DIRECTION('ref_axis',(1.,0.,0.));
#19490=DIRECTION('center_axis',(0.,0.,-1.));
#19491=DIRECTION('ref_axis',(1.,0.,0.));
#19492=DIRECTION('',(0.,0.,-1.));
#19493=DIRECTION('center_axis',(0.,0.,-1.));
#19494=DIRECTION('ref_axis',(1.,0.,0.));
#19495=DIRECTION('center_axis',(0.,0.,-1.));
#19496=DIRECTION('ref_axis',(1.,0.,0.));
#19497=DIRECTION('center_axis',(0.,0.,-1.));
#19498=DIRECTION('ref_axis',(1.,0.,0.));
#19499=DIRECTION('center_axis',(0.,0.,-1.));
#19500=DIRECTION('ref_axis',(1.,0.,0.));
#19501=DIRECTION('center_axis',(0.,0.,-1.));
#19502=DIRECTION('ref_axis',(1.,0.,0.));
#19503=DIRECTION('center_axis',(0.,0.,-1.));
#19504=DIRECTION('ref_axis',(1.,0.,0.));
#19505=DIRECTION('center_axis',(0.,0.,-1.));
#19506=DIRECTION('ref_axis',(1.,0.,0.));
#19507=DIRECTION('center_axis',(0.,0.,-1.));
#19508=DIRECTION('ref_axis',(1.,0.,0.));
#19509=DIRECTION('center_axis',(0.,0.,-1.));
#19510=DIRECTION('ref_axis',(1.,0.,0.));
#19511=DIRECTION('center_axis',(0.,0.,-1.));
#19512=DIRECTION('ref_axis',(1.,0.,0.));
#19513=DIRECTION('center_axis',(0.,0.,-1.));
#19514=DIRECTION('ref_axis',(1.,0.,0.));
#19515=DIRECTION('center_axis',(0.,0.,-1.));
#19516=DIRECTION('ref_axis',(1.,0.,0.));
#19517=DIRECTION('center_axis',(0.,0.,1.));
#19518=DIRECTION('ref_axis',(1.,0.,0.));
#19519=DIRECTION('center_axis',(0.,0.,1.));
#19520=DIRECTION('ref_axis',(1.,0.,0.));
#19521=DIRECTION('center_axis',(0.,0.,1.));
#19522=DIRECTION('ref_axis',(0.,-1.,0.));
#19523=DIRECTION('center_axis',(0.,0.,1.));
#19524=DIRECTION('ref_axis',(1.,0.,0.));
#19525=DIRECTION('center_axis',(0.,0.,1.));
#19526=DIRECTION('ref_axis',(0.,-1.,0.));
#19527=DIRECTION('center_axis',(0.,1.,0.));
#19528=DIRECTION('ref_axis',(-1.,0.,0.));
#19529=DIRECTION('center_axis',(0.,0.,1.));
#19530=DIRECTION('ref_axis',(1.,0.,0.));
#19531=DIRECTION('center_axis',(0.,0.,1.));
#19532=DIRECTION('ref_axis',(1.,0.,0.));
#19533=DIRECTION('center_axis',(0.,0.,1.));
#19534=DIRECTION('ref_axis',(0.,-1.,0.));
#19535=DIRECTION('center_axis',(6.12323399573677E-17,0.,1.));
#19536=DIRECTION('ref_axis',(1.,0.,0.));
#19537=DIRECTION('center_axis',(0.,0.,1.));
#19538=DIRECTION('ref_axis',(0.,-1.,0.));
#19539=DIRECTION('center_axis',(0.,1.,0.));
#19540=DIRECTION('ref_axis',(-1.,0.,0.));
#19541=DIRECTION('center_axis',(0.,0.,1.));
#19542=DIRECTION('ref_axis',(0.,-1.,0.));
#19543=DIRECTION('center_axis',(0.,0.,1.));
#19544=DIRECTION('ref_axis',(1.,0.,0.));
#19545=DIRECTION('center_axis',(0.,0.,1.));
#19546=DIRECTION('ref_axis',(1.,0.,0.));
#19547=DIRECTION('center_axis',(0.,0.,1.));
#19548=DIRECTION('ref_axis',(0.,-1.,0.));
#19549=DIRECTION('center_axis',(0.,0.,1.));
#19550=DIRECTION('ref_axis',(1.,0.,0.));
#19551=DIRECTION('center_axis',(0.,0.,1.));
#19552=DIRECTION('ref_axis',(0.,-1.,0.));
#19553=DIRECTION('center_axis',(0.,1.,0.));
#19554=DIRECTION('ref_axis',(-1.,0.,0.));
#19555=DIRECTION('center_axis',(0.,0.,1.));
#19556=DIRECTION('ref_axis',(1.,0.,0.));
#19557=DIRECTION('center_axis',(0.,0.,1.));
#19558=DIRECTION('ref_axis',(1.,0.,0.));
#19559=DIRECTION('center_axis',(0.,0.,1.));
#19560=DIRECTION('ref_axis',(0.,-1.,0.));
#19561=DIRECTION('center_axis',(0.,0.,1.));
#19562=DIRECTION('ref_axis',(1.,0.,0.));
#19563=DIRECTION('center_axis',(0.,0.,1.));
#19564=DIRECTION('ref_axis',(0.,-1.,0.));
#19565=DIRECTION('center_axis',(0.,1.,0.));
#19566=DIRECTION('ref_axis',(-1.,0.,0.));
#19567=DIRECTION('center_axis',(0.,0.,1.));
#19568=DIRECTION('ref_axis',(1.,0.,0.));
#19569=DIRECTION('center_axis',(0.,0.,1.));
#19570=DIRECTION('ref_axis',(1.,0.,0.));
#19571=DIRECTION('center_axis',(0.,0.,1.));
#19572=DIRECTION('ref_axis',(0.,-1.,0.));
#19573=DIRECTION('center_axis',(0.,0.,1.));
#19574=DIRECTION('ref_axis',(1.,0.,0.));
#19575=DIRECTION('center_axis',(0.,0.,1.));
#19576=DIRECTION('ref_axis',(0.,-1.,0.));
#19577=DIRECTION('center_axis',(-1.22464679914735E-16,1.,0.));
#19578=DIRECTION('ref_axis',(-1.,-1.22464679914735E-16,0.));
#19579=DIRECTION('center_axis',(0.,0.,1.));
#19580=DIRECTION('ref_axis',(1.,0.,0.));
#19581=DIRECTION('center_axis',(0.,0.,1.));
#19582=DIRECTION('ref_axis',(1.,0.,0.));
#19583=DIRECTION('center_axis',(0.,0.,1.));
#19584=DIRECTION('ref_axis',(0.,-1.,0.));
#19585=DIRECTION('center_axis',(0.,0.,1.));
#19586=DIRECTION('ref_axis',(1.,0.,0.));
#19587=DIRECTION('center_axis',(0.,0.,1.));
#19588=DIRECTION('ref_axis',(0.,-1.,0.));
#19589=DIRECTION('center_axis',(0.,1.,0.));
#19590=DIRECTION('ref_axis',(-1.,0.,0.));
#19591=DIRECTION('center_axis',(0.,0.,1.));
#19592=DIRECTION('ref_axis',(1.,0.,0.));
#19593=DIRECTION('center_axis',(0.,0.,1.));
#19594=DIRECTION('ref_axis',(1.,0.,0.));
#19595=DIRECTION('center_axis',(0.,0.,1.));
#19596=DIRECTION('ref_axis',(0.,-1.,0.));
#19597=DIRECTION('center_axis',(0.,0.,1.));
#19598=DIRECTION('ref_axis',(1.,0.,0.));
#19599=DIRECTION('center_axis',(0.,0.,1.));
#19600=DIRECTION('ref_axis',(0.,-1.,0.));
#19601=DIRECTION('center_axis',(0.,1.,0.));
#19602=DIRECTION('ref_axis',(-1.,0.,0.));
#19603=DIRECTION('center_axis',(0.,0.,1.));
#19604=DIRECTION('ref_axis',(1.,0.,0.));
#19605=DIRECTION('center_axis',(0.,0.,1.));
#19606=DIRECTION('ref_axis',(1.,0.,0.));
#19607=DIRECTION('center_axis',(0.,0.,1.));
#19608=DIRECTION('ref_axis',(0.,-1.,0.));
#19609=DIRECTION('center_axis',(0.,0.,1.));
#19610=DIRECTION('ref_axis',(0.,-1.,0.));
#19611=DIRECTION('center_axis',(6.12323399573677E-17,0.,1.));
#19612=DIRECTION('ref_axis',(1.,0.,0.));
#19613=DIRECTION('center_axis',(0.,0.,1.));
#19614=DIRECTION('ref_axis',(0.,-1.,0.));
#19615=DIRECTION('center_axis',(0.,1.,0.));
#19616=DIRECTION('ref_axis',(-1.,0.,0.));
#19617=DIRECTION('center_axis',(0.,0.,1.));
#19618=DIRECTION('ref_axis',(1.,0.,0.));
#19619=DIRECTION('center_axis',(0.,0.,1.));
#19620=DIRECTION('ref_axis',(1.,0.,0.));
#19621=DIRECTION('center_axis',(0.,0.,1.));
#19622=DIRECTION('ref_axis',(0.,-1.,0.));
#19623=DIRECTION('center_axis',(0.,0.,1.));
#19624=DIRECTION('ref_axis',(1.,0.,0.));
#19625=DIRECTION('center_axis',(0.,0.,1.));
#19626=DIRECTION('ref_axis',(0.,-1.,0.));
#19627=DIRECTION('center_axis',(0.,1.,0.));
#19628=DIRECTION('ref_axis',(-1.,0.,0.));
#19629=DIRECTION('center_axis',(0.,0.,1.));
#19630=DIRECTION('ref_axis',(1.,0.,0.));
#19631=DIRECTION('center_axis',(0.,0.,1.));
#19632=DIRECTION('ref_axis',(1.,0.,0.));
#19633=DIRECTION('center_axis',(0.,0.,1.));
#19634=DIRECTION('ref_axis',(0.,-1.,0.));
#19635=DIRECTION('center_axis',(0.,0.,1.));
#19636=DIRECTION('ref_axis',(1.,0.,0.));
#19637=DIRECTION('center_axis',(0.,0.,1.));
#19638=DIRECTION('ref_axis',(0.,-1.,0.));
#19639=DIRECTION('center_axis',(0.,1.,0.));
#19640=DIRECTION('ref_axis',(-1.,0.,0.));
#19641=DIRECTION('center_axis',(0.,0.,1.));
#19642=DIRECTION('ref_axis',(1.,0.,0.));
#19643=DIRECTION('center_axis',(0.,0.,1.));
#19644=DIRECTION('ref_axis',(1.,0.,0.));
#19645=DIRECTION('center_axis',(0.,0.,1.));
#19646=DIRECTION('ref_axis',(0.,-1.,0.));
#19647=DIRECTION('center_axis',(0.,0.,1.));
#19648=DIRECTION('ref_axis',(1.,0.,0.));
#19649=DIRECTION('center_axis',(0.,0.,1.));
#19650=DIRECTION('ref_axis',(0.,-1.,0.));
#19651=DIRECTION('center_axis',(-1.22464679914735E-16,1.,0.));
#19652=DIRECTION('ref_axis',(-1.,-1.22464679914735E-16,0.));
#19653=DIRECTION('center_axis',(0.,0.,1.));
#19654=DIRECTION('ref_axis',(1.,0.,0.));
#19655=DIRECTION('center_axis',(0.,0.,1.));
#19656=DIRECTION('ref_axis',(1.,0.,0.));
#19657=DIRECTION('',(0.,0.,-1.));
#19658=DIRECTION('center_axis',(0.,0.,1.));
#19659=DIRECTION('ref_axis',(1.,0.,0.));
#19660=DIRECTION('center_axis',(0.,0.,1.));
#19661=DIRECTION('ref_axis',(1.,0.,0.));
#19662=DIRECTION('center_axis',(0.,0.,1.));
#19663=DIRECTION('ref_axis',(1.,0.,0.));
#60430=CARTESIAN_POINT('',(0.,0.,0.));
#60431=CARTESIAN_POINT('Origin',(25.9807621135332,-15.,0.));
#60432=CARTESIAN_POINT('',(24.3419428085142,-20.771851634051,0.));
#60433=CARTESIAN_POINT('',(30.1599226029865,-10.6948150326157,0.));
#60434=CARTESIAN_POINT('Ctrl Pts',(24.3419428085141,-20.771851634051,-5.55111512312578E-16));
#60435=CARTESIAN_POINT('Ctrl Pts',(24.3419428085141,-20.771851634051,0.650190448083162));
#60436=CARTESIAN_POINT('Ctrl Pts',(24.4227996788253,-20.6782577017963,1.34576815070429));
#60437=CARTESIAN_POINT('Ctrl Pts',(24.7453933436892,-20.2911063999427,2.63799288444813));
#60438=CARTESIAN_POINT('Ctrl Pts',(24.9861795488087,-19.9970150157524,3.23471700046071));
#60439=CARTESIAN_POINT('Ctrl Pts',(25.3750265832533,-19.4973595993855,3.93620747216805));
#60440=CARTESIAN_POINT('Ctrl Pts',(25.5173253431967,-19.3113833049334,4.15945687249389));
#60441=CARTESIAN_POINT('Ctrl Pts',(25.8180939601395,-18.9073912038163,4.56176656225471));
#60442=CARTESIAN_POINT('Ctrl Pts',(25.9764367690932,-18.6893185292651,4.74086471477472));
#60443=CARTESIAN_POINT('Ctrl Pts',(26.3690354996372,-18.1343047842461,5.12459397949762));
#60444=CARTESIAN_POINT('Ctrl Pts',(26.6450813997796,-17.7284768246621,5.32832509625205));
#60445=CARTESIAN_POINT('Ctrl Pts',(27.1956249100491,-16.8717882618769,5.59441429610713));
#60446=CARTESIAN_POINT('Ctrl Pts',(27.4698694309609,-16.4207904682926,5.65685424949238));
#60447=CARTESIAN_POINT('Ctrl Pts',(27.9557564112432,-15.5792095317074,5.65685424949238));
#60448=CARTESIAN_POINT('Ctrl Pts',(28.2092096970821,-15.116207912957,5.59441429610713));
#60449=CARTESIAN_POINT('Ctrl Pts',(28.6758520004508,-14.2110789657823,5.32832509625205));
#60450=CARTESIAN_POINT('Ctrl Pts',(28.8892863729454,-13.7691022238565,5.12459397949763));
#60451=CARTESIAN_POINT('Ctrl Pts',(29.1736430103094,-13.1515948772024,4.74086471477473));
#60452=CARTESIAN_POINT('Ctrl Pts',(29.2833280818651,-12.9054296448663,4.56176656225472));
#60453=CARTESIAN_POINT('Ctrl Pts',(29.4828111958893,-12.4429603313742,4.15945687249389));
#60454=CARTESIAN_POINT('Ctrl Pts',(29.5727220114149,-12.2267378431101,3.93620747216806));
#60455=CARTESIAN_POINT('Ctrl Pts',(29.8110127779048,-11.6401587249113,3.23471700046071));
#60456=CARTESIAN_POINT('Ctrl Pts',(29.945310285088,-11.2845860623018,2.63799288444813));
#60457=CARTESIAN_POINT('Ctrl Pts',(30.1192963151694,-10.811636102503,1.34576815070429));
#60458=CARTESIAN_POINT('Ctrl Pts',(30.1599226029865,-10.6948150326157,0.650190448083163));
#60459=CARTESIAN_POINT('Ctrl Pts',(30.1599226029865,-10.6948150326157,1.38777878078145E-16));
#60460=CARTESIAN_POINT('',(21.0673540166964,-18.4436057953749,0.));
#60461=CARTESIAN_POINT('Origin',(25.9807621135332,-15.,0.));
#60462=CARTESIAN_POINT('',(23.6431808351666,-14.9999999999269,5.52591293516556));
#60463=CARTESIAN_POINT('Ctrl Pts',(23.6431808351666,-14.9999999998537,5.52591293516556));
#60464=CARTESIAN_POINT('Ctrl Pts',(23.6009406541951,-15.0665794823356,5.50804442051787));
#60465=CARTESIAN_POINT('Ctrl Pts',(23.5585526426266,-15.1327690152579,5.48833637748936));
#60466=CARTESIAN_POINT('Ctrl Pts',(23.2618588909767,-15.5918378185285,5.3379209922756));
#60467=CARTESIAN_POINT('Ctrl Pts',(23.0071885556824,-15.9630484519639,5.14122028307955));
#60468=CARTESIAN_POINT('Ctrl Pts',(22.5419616872921,-16.6141770101942,4.66899487999358));
#60469=CARTESIAN_POINT('Ctrl Pts',(22.3089325549727,-16.9242282724357,4.36544996647721));
#60470=CARTESIAN_POINT('Ctrl Pts',(21.8870655758732,-17.4663772648075,3.66070649008719));
#60471=CARTESIAN_POINT('Ctrl Pts',(21.6983404251917,-17.6986070028546,3.25954202901027));
#60472=CARTESIAN_POINT('Ctrl Pts',(21.2342115445438,-18.2576809083209,1.96027825599731));
#60473=CARTESIAN_POINT('Ctrl Pts',(21.0673540166964,-18.4436057953749,0.960060375520683));
#60474=CARTESIAN_POINT('Ctrl Pts',(21.0673540166964,-18.4436057953749,0.));
#60475=CARTESIAN_POINT('',(25.9807621135332,-15.,6.));
#60476=CARTESIAN_POINT('Origin',(25.9807621135332,-15.,0.));
#60477=CARTESIAN_POINT('',(26.5063081645287,-9.02306087129181,0.));
#60478=CARTESIAN_POINT('Ctrl Pts',(26.5063081645287,-9.02306087129183,-2.77555756156289E-16));
#60479=CARTESIAN_POINT('Ctrl Pts',(26.5063081645287,-9.02306087129183,0.960060375520683));
#60480=CARTESIAN_POINT('Ctrl Pts',(26.428721253068,-9.26052617274731,1.96027825599731));
#60481=CARTESIAN_POINT('Ctrl Pts',(26.1766134886651,-9.94201052675154,3.25954202901027));
#60482=CARTESIAN_POINT('Ctrl Pts',(26.0698592113429,-10.2215661705984,3.6607064900872));
#60483=CARTESIAN_POINT('Ctrl Pts',(25.8112779008625,-10.8579881877023,4.36544996647721));
#60484=CARTESIAN_POINT('Ctrl Pts',(25.6592801974456,-11.2148229672334,4.66899487999358));
#60485=CARTESIAN_POINT('Ctrl Pts',(25.3279997590838,-11.9432855328977,5.14122028307955));
#60486=CARTESIAN_POINT('Ctrl Pts',(25.1338570880209,-12.3494418295706,5.3379209922756));
#60487=CARTESIAN_POINT('Ctrl Pts',(24.7066441580527,-13.1833691308415,5.59576473572533));
#60488=CARTESIAN_POINT('Ctrl Pts',(24.4732931529197,-13.6110128306156,5.65685424949238));
#60489=CARTESIAN_POINT('Ctrl Pts',(24.0615711505723,-14.3241362572753,5.65685424949238));
#60490=CARTESIAN_POINT('Ctrl Pts',(23.8543046840289,-14.6672240440326,5.61522291204339));
#60491=CARTESIAN_POINT('Ctrl Pts',(23.6431808351666,-14.9999999998537,5.52591293516556));
#60492=CARTESIAN_POINT('Origin',(25.9807621135332,-15.,0.));
#60493=CARTESIAN_POINT('Origin',(0.,0.,0.));
#60494=CARTESIAN_POINT('',(-28.,-3.42901103761259E-15,8.));
#60495=CARTESIAN_POINT('Origin',(0.,0.,8.));
#60496=CARTESIAN_POINT('',(-28.,8.96068962095847E-17,5.65685424949238));
#60497=CARTESIAN_POINT('',(-28.,-3.42901103761259E-15,0.));
#60498=CARTESIAN_POINT('',(-27.4666666666667,5.43895414783232,0.));
#60499=CARTESIAN_POINT('Ctrl Pts',(-28.,3.88578058618805E-15,5.65685424949238));
#60500=CARTESIAN_POINT('Ctrl Pts',(-28.,0.449163693910781,5.65685424949238));
#60501=CARTESIAN_POINT('Ctrl Pts',(-27.9882660485567,0.936189504250082,
5.59576473572533));
#60502=CARTESIAN_POINT('Ctrl Pts',(-27.941279648099,1.8719981970442,5.3379209922756));
#60503=CARTESIAN_POINT('Ctrl Pts',(-27.9063339848615,2.32081120340133,5.14122028307955));
#60504=CARTESIAN_POINT('Ctrl Pts',(-27.8289999774276,3.11731851015347,4.66899487999359));
#60505=CARTESIAN_POINT('Ctrl Pts',(-27.7822164601379,3.50234534588973,4.36544996647722));
#60506=CARTESIAN_POINT('Ctrl Pts',(-27.6879434354058,4.18279363546963,3.6607064900872));
#60507=CARTESIAN_POINT('Ctrl Pts',(-27.6406175296061,4.47827306347342,3.25954202901027));
#60508=CARTESIAN_POINT('Ctrl Pts',(-27.5182070810682,5.19450970852415,1.96027825599731));
#60509=CARTESIAN_POINT('Ctrl Pts',(-27.4666666666667,5.43895414783231,0.960060375520684));
#60510=CARTESIAN_POINT('Ctrl Pts',(-27.4666666666667,5.43895414783231,-5.55111512312578E-16));
#60511=CARTESIAN_POINT('',(-26.5063081645287,9.0230608712918,0.));
#60512=CARTESIAN_POINT('Origin',(0.,0.,0.));
#60513=CARTESIAN_POINT('',(-21.0673540166964,18.4436057953749,0.));
#60514=CARTESIAN_POINT('Ctrl Pts',(-26.5063081645287,9.02306087129181,-5.55111512312578E-16));
#60515=CARTESIAN_POINT('Ctrl Pts',(-26.5063081645287,9.02306087129181,0.960060375520683));
#60516=CARTESIAN_POINT('Ctrl Pts',(-26.428721253068,9.2605261727473,1.96027825599731));
#60517=CARTESIAN_POINT('Ctrl Pts',(-26.1766134886651,9.94201052675152,3.25954202901027));
#60518=CARTESIAN_POINT('Ctrl Pts',(-26.0698592113429,10.2215661705984,3.6607064900872));
#60519=CARTESIAN_POINT('Ctrl Pts',(-25.8112779008625,10.8579881877022,4.36544996647722));
#60520=CARTESIAN_POINT('Ctrl Pts',(-25.6592801974456,11.2148229672334,4.66899487999358));
#60521=CARTESIAN_POINT('Ctrl Pts',(-25.3279997590838,11.9432855328977,5.14122028307955));
#60522=CARTESIAN_POINT('Ctrl Pts',(-25.1338570880209,12.3494418295705,5.3379209922756));
#60523=CARTESIAN_POINT('Ctrl Pts',(-24.7066441580527,13.1833691308414,5.59576473572533));
#60524=CARTESIAN_POINT('Ctrl Pts',(-24.4732931529197,13.6110128306156,5.65685424949238));
#60525=CARTESIAN_POINT('Ctrl Pts',(-24.0241294590089,14.3889871693844,5.65685424949238));
#60526=CARTESIAN_POINT('Ctrl Pts',(-23.7704546538026,14.8048969177153,5.59576473572533));
#60527=CARTESIAN_POINT('Ctrl Pts',(-23.2618588909767,15.5918378185284,5.3379209922756));
#60528=CARTESIAN_POINT('Ctrl Pts',(-23.0071885556824,15.9630484519638,5.14122028307955));
#60529=CARTESIAN_POINT('Ctrl Pts',(-22.5419616872921,16.6141770101942,4.66899487999358));
#60530=CARTESIAN_POINT('Ctrl Pts',(-22.3089325549727,16.9242282724357,4.36544996647721));
#60531=CARTESIAN_POINT('Ctrl Pts',(-21.8870655758732,17.4663772648075,3.66070649008719));
#60532=CARTESIAN_POINT('Ctrl Pts',(-21.6983404251917,17.6986070028546,3.25954202901027));
#60533=CARTESIAN_POINT('Ctrl Pts',(-21.2342115445438,18.2576809083209,1.96027825599731));
#60534=CARTESIAN_POINT('Ctrl Pts',(-21.0673540166964,18.4436057953748,0.960060375520683));
#60535=CARTESIAN_POINT('Ctrl Pts',(-21.0673540166964,18.4436057953748,-2.77555756156289E-16));
#60536=CARTESIAN_POINT('',(-18.4436057953749,21.0673540166964,0.));
#60537=CARTESIAN_POINT('Origin',(0.,0.,0.));
#60538=CARTESIAN_POINT('',(-9.0230608712918,26.5063081645287,0.));
#60539=CARTESIAN_POINT('Ctrl Pts',(-18.4436057953748,21.0673540166964,-2.77555756156289E-16));
#60540=CARTESIAN_POINT('Ctrl Pts',(-18.4436057953748,21.0673540166964,0.960060375520684));
#60541=CARTESIAN_POINT('Ctrl Pts',(-18.2576809083209,21.2342115445438,1.96027825599731));
#60542=CARTESIAN_POINT('Ctrl Pts',(-17.6986070028546,21.6983404251917,3.25954202901027));
#60543=CARTESIAN_POINT('Ctrl Pts',(-17.4663772648075,21.8870655758732,3.6607064900872));
#60544=CARTESIAN_POINT('Ctrl Pts',(-16.9242282724357,22.3089325549727,4.36544996647722));
#60545=CARTESIAN_POINT('Ctrl Pts',(-16.6141770101941,22.5419616872921,4.66899487999358));
#60546=CARTESIAN_POINT('Ctrl Pts',(-15.9630484519638,23.0071885556824,5.14122028307955));
#60547=CARTESIAN_POINT('Ctrl Pts',(-15.5918378185284,23.2618588909768,5.3379209922756));
#60548=CARTESIAN_POINT('Ctrl Pts',(-14.8048969177153,23.7704546538026,5.59576473572533));
#60549=CARTESIAN_POINT('Ctrl Pts',(-14.3889871693844,24.0241294590089,5.65685424949238));
#60550=CARTESIAN_POINT('Ctrl Pts',(-13.6110128306156,24.4732931529197,5.65685424949238));
#60551=CARTESIAN_POINT('Ctrl Pts',(-13.1833691308414,24.7066441580527,5.59576473572533));
#60552=CARTESIAN_POINT('Ctrl Pts',(-12.3494418295705,25.1338570880209,5.3379209922756));
#60553=CARTESIAN_POINT('Ctrl Pts',(-11.9432855328977,25.3279997590838,5.14122028307955));
#60554=CARTESIAN_POINT('Ctrl Pts',(-11.2148229672334,25.6592801974456,4.66899487999358));
#60555=CARTESIAN_POINT('Ctrl Pts',(-10.8579881877022,25.8112779008625,4.36544996647721));
#60556=CARTESIAN_POINT('Ctrl Pts',(-10.2215661705984,26.0698592113429,3.6607064900872));
#60557=CARTESIAN_POINT('Ctrl Pts',(-9.94201052675152,26.1766134886651,3.25954202901027));
#60558=CARTESIAN_POINT('Ctrl Pts',(-9.26052617274729,26.428721253068,1.96027825599731));
#60559=CARTESIAN_POINT('Ctrl Pts',(-9.02306087129181,26.5063081645287,0.960060375520683));
#60560=CARTESIAN_POINT('Ctrl Pts',(-9.02306087129181,26.5063081645287,-2.77555756156289E-16));
#60561=CARTESIAN_POINT('',(-5.43895414783229,27.4666666666667,0.));
#60562=CARTESIAN_POINT('Origin',(0.,0.,0.));
#60563=CARTESIAN_POINT('',(5.4389541478323,27.4666666666667,0.));
#60564=CARTESIAN_POINT('Ctrl Pts',(-5.4389541478323,27.4666666666667,2.77555756156289E-16));
#60565=CARTESIAN_POINT('Ctrl Pts',(-5.4389541478323,27.4666666666667,0.960060375520684));
#60566=CARTESIAN_POINT('Ctrl Pts',(-5.19450970852415,27.5182070810682,1.96027825599731));
#60567=CARTESIAN_POINT('Ctrl Pts',(-4.47827306347342,27.6406175296061,3.25954202901027));
#60568=CARTESIAN_POINT('Ctrl Pts',(-4.18279363546962,27.6879434354058,3.6607064900872));
#60569=CARTESIAN_POINT('Ctrl Pts',(-3.50234534588973,27.7822164601379,4.36544996647721));
#60570=CARTESIAN_POINT('Ctrl Pts',(-3.11731851015347,27.8289999774276,4.66899487999358));
#60571=CARTESIAN_POINT('Ctrl Pts',(-2.32081120340133,27.9063339848615,5.14122028307955));
#60572=CARTESIAN_POINT('Ctrl Pts',(-1.8719981970442,27.941279648099,5.3379209922756));
#60573=CARTESIAN_POINT('Ctrl Pts',(-0.936189504250081,27.9882660485567,
5.59576473572533));
#60574=CARTESIAN_POINT('Ctrl Pts',(-0.449163693910777,28.,5.65685424949238));
#60575=CARTESIAN_POINT('Ctrl Pts',(0.449163693910781,28.,5.65685424949238));
#60576=CARTESIAN_POINT('Ctrl Pts',(0.936189504250085,27.9882660485567,5.59576473572533));
#60577=CARTESIAN_POINT('Ctrl Pts',(1.8719981970442,27.941279648099,5.3379209922756));
#60578=CARTESIAN_POINT('Ctrl Pts',(2.32081120340133,27.9063339848615,5.14122028307955));
#60579=CARTESIAN_POINT('Ctrl Pts',(3.11731851015347,27.8289999774276,4.66899487999358));
#60580=CARTESIAN_POINT('Ctrl Pts',(3.50234534588973,27.7822164601379,4.36544996647721));
#60581=CARTESIAN_POINT('Ctrl Pts',(4.18279363546963,27.6879434354058,3.6607064900872));
#60582=CARTESIAN_POINT('Ctrl Pts',(4.47827306347342,27.6406175296061,3.25954202901027));
#60583=CARTESIAN_POINT('Ctrl Pts',(5.19450970852415,27.5182070810682,1.96027825599731));
#60584=CARTESIAN_POINT('Ctrl Pts',(5.4389541478323,27.4666666666667,0.960060375520683));
#60585=CARTESIAN_POINT('Ctrl Pts',(5.4389541478323,27.4666666666667,2.77555756156289E-16));
#60586=CARTESIAN_POINT('',(9.0230608712918,26.5063081645287,0.));
#60587=CARTESIAN_POINT('Origin',(0.,0.,0.));
#60588=CARTESIAN_POINT('',(10.4403065089456,25.9807621135261,3.89989682781948));
#60589=CARTESIAN_POINT('Ctrl Pts',(9.02306087129182,26.5063081645287,0.));
#60590=CARTESIAN_POINT('Ctrl Pts',(9.02306087129182,26.5063081645287,0.960060375520684));
#60591=CARTESIAN_POINT('Ctrl Pts',(9.2605261727473,26.428721253068,1.96027825599731));
#60592=CARTESIAN_POINT('Ctrl Pts',(9.9180326009165,26.1854838629323,3.21382762602157));
#60593=CARTESIAN_POINT('Ctrl Pts',(10.1630550776949,26.0921749315747,3.57573913794424));
#60594=CARTESIAN_POINT('Ctrl Pts',(10.4403065089456,25.9807621135191,3.89989682781948));
#60595=CARTESIAN_POINT('',(18.4436057953749,21.0673540166964,0.));
#60596=CARTESIAN_POINT('Ctrl Pts',(10.4403065089456,25.9807621135191,3.89989682781948));
#60597=CARTESIAN_POINT('Ctrl Pts',(10.4730252750948,25.9676141563614,3.93815105649065));
#60598=CARTESIAN_POINT('Ctrl Pts',(10.5061885578498,25.9542157736402,3.97588378637688));
#60599=CARTESIAN_POINT('Ctrl Pts',(10.8579881877023,25.8112779008625,4.36544996647722));
#60600=CARTESIAN_POINT('Ctrl Pts',(11.2148229672334,25.6592801974456,4.66899487999358));
#60601=CARTESIAN_POINT('Ctrl Pts',(11.9432855328977,25.3279997590838,5.14122028307955));
#60602=CARTESIAN_POINT('Ctrl Pts',(12.3494418295706,25.1338570880209,5.3379209922756));
#60603=CARTESIAN_POINT('Ctrl Pts',(13.1833691308414,24.7066441580527,5.59576473572533));
#60604=CARTESIAN_POINT('Ctrl Pts',(13.6110128306156,24.4732931529197,5.65685424949238));
#60605=CARTESIAN_POINT('Ctrl Pts',(14.3889871693844,24.0241294590089,5.65685424949238));
#60606=CARTESIAN_POINT('Ctrl Pts',(14.8048969177153,23.7704546538026,5.59576473572533));
#60607=CARTESIAN_POINT('Ctrl Pts',(15.5918378185284,23.2618588909767,5.3379209922756));
#60608=CARTESIAN_POINT('Ctrl Pts',(15.9630484519639,23.0071885556824,5.14122028307955));
#60609=CARTESIAN_POINT('Ctrl Pts',(16.6141770101942,22.5419616872921,4.66899487999358));
#60610=CARTESIAN_POINT('Ctrl Pts',(16.9242282724357,22.3089325549727,4.36544996647722));
#60611=CARTESIAN_POINT('Ctrl Pts',(17.4663772648075,21.8870655758732,3.6607064900872));
#60612=CARTESIAN_POINT('Ctrl Pts',(17.6986070028546,21.6983404251917,3.25954202901027));
#60613=CARTESIAN_POINT('Ctrl Pts',(18.2576809083209,21.2342115445438,1.96027825599731));
#60614=CARTESIAN_POINT('Ctrl Pts',(18.4436057953749,21.0673540166964,0.960060375520683));
#60615=CARTESIAN_POINT('Ctrl Pts',(18.4436057953749,21.0673540166964,-2.77555756156289E-16));
#60616=CARTESIAN_POINT('',(21.0673540166964,18.4436057953749,0.));
#60617=CARTESIAN_POINT('Origin',(0.,0.,0.));
#60618=CARTESIAN_POINT('',(23.6431808351666,14.9999999999269,5.52591293516556));
#60619=CARTESIAN_POINT('Ctrl Pts',(21.0673540166964,18.4436057953749,-2.77555756156289E-16));
#60620=CARTESIAN_POINT('Ctrl Pts',(21.0673540166964,18.4436057953749,0.960060375520684));
#60621=CARTESIAN_POINT('Ctrl Pts',(21.2342115445438,18.2576809083209,1.96027825599731));
#60622=CARTESIAN_POINT('Ctrl Pts',(21.6983404251917,17.6986070028546,3.25954202901027));
#60623=CARTESIAN_POINT('Ctrl Pts',(21.8870655758732,17.4663772648075,3.6607064900872));
#60624=CARTESIAN_POINT('Ctrl Pts',(22.3089325549727,16.9242282724357,4.36544996647722));
#60625=CARTESIAN_POINT('Ctrl Pts',(22.5419616872921,16.6141770101941,4.66899487999358));
#60626=CARTESIAN_POINT('Ctrl Pts',(23.0071885556824,15.9630484519638,5.14122028307955));
#60627=CARTESIAN_POINT('Ctrl Pts',(23.2618588909767,15.5918378185284,5.3379209922756));
#60628=CARTESIAN_POINT('Ctrl Pts',(23.5585526426266,15.1327690152579,5.48833637748937));
#60629=CARTESIAN_POINT('Ctrl Pts',(23.6009406541952,15.0665794823355,5.50804442051787));
#60630=CARTESIAN_POINT('Ctrl Pts',(23.6431808351666,14.9999999998537,5.52591293516556));
#60631=CARTESIAN_POINT('',(26.5063081645287,9.0230608712918,0.));
#60632=CARTESIAN_POINT('Ctrl Pts',(23.6431808351666,14.9999999998537,5.52591293516556));
#60633=CARTESIAN_POINT('Ctrl Pts',(23.8543046840289,14.6672240440326,5.61522291204339));
#60634=CARTESIAN_POINT('Ctrl Pts',(24.0615711505723,14.3241362572753,5.65685424949238));
#60635=CARTESIAN_POINT('Ctrl Pts',(24.4732931529197,13.6110128306156,5.65685424949238));
#60636=CARTESIAN_POINT('Ctrl Pts',(24.7066441580527,13.1833691308414,5.59576473572533));
#60637=CARTESIAN_POINT('Ctrl Pts',(25.1338570880209,12.3494418295705,5.3379209922756));
#60638=CARTESIAN_POINT('Ctrl Pts',(25.3279997590838,11.9432855328977,5.14122028307955));
#60639=CARTESIAN_POINT('Ctrl Pts',(25.6592801974456,11.2148229672334,4.66899487999358));
#60640=CARTESIAN_POINT('Ctrl Pts',(25.8112779008625,10.8579881877022,4.36544996647722));
#60641=CARTESIAN_POINT('Ctrl Pts',(26.0698592113429,10.2215661705984,3.6607064900872));
#60642=CARTESIAN_POINT('Ctrl Pts',(26.1766134886651,9.94201052675152,3.25954202901027));
#60643=CARTESIAN_POINT('Ctrl Pts',(26.428721253068,9.2605261727473,1.96027825599731));
#60644=CARTESIAN_POINT('Ctrl Pts',(26.5063081645287,9.02306087129181,0.960060375520683));
#60645=CARTESIAN_POINT('Ctrl Pts',(26.5063081645287,9.02306087129181,-2.77555756156289E-16));
#60646=CARTESIAN_POINT('',(27.4666666666667,5.43895414783232,0.));
#60647=CARTESIAN_POINT('Origin',(0.,0.,0.));
#60648=CARTESIAN_POINT('',(28.,-2.6124255799288E-16,5.65685424949238));
#60649=CARTESIAN_POINT('Ctrl Pts',(27.4666666666667,5.4389541478323,-2.77555756156289E-16));
#60650=CARTESIAN_POINT('Ctrl Pts',(27.4666666666667,5.4389541478323,0.960060375520684));
#60651=CARTESIAN_POINT('Ctrl Pts',(27.5182070810682,5.19450970852415,1.96027825599731));
#60652=CARTESIAN_POINT('Ctrl Pts',(27.6406175296061,4.47827306347342,3.25954202901027));
#60653=CARTESIAN_POINT('Ctrl Pts',(27.6879434354058,4.18279363546963,3.6607064900872));
#60654=CARTESIAN_POINT('Ctrl Pts',(27.7822164601379,3.50234534588973,4.36544996647722));
#60655=CARTESIAN_POINT('Ctrl Pts',(27.8289999774276,3.11731851015347,4.66899487999358));
#60656=CARTESIAN_POINT('Ctrl Pts',(27.9063339848615,2.32081120340133,5.14122028307955));
#60657=CARTESIAN_POINT('Ctrl Pts',(27.941279648099,1.8719981970442,5.3379209922756));
#60658=CARTESIAN_POINT('Ctrl Pts',(27.9882660485567,0.936189504250083,5.59576473572533));
#60659=CARTESIAN_POINT('Ctrl Pts',(28.,0.449163693910779,5.65685424949238));
#60660=CARTESIAN_POINT('Ctrl Pts',(28.,-1.38777878078145E-16,5.65685424949238));
#60661=CARTESIAN_POINT('',(27.4666666666667,-5.43895414783232,0.));
#60662=CARTESIAN_POINT('Ctrl Pts',(28.,0.,5.65685424949238));
#60663=CARTESIAN_POINT('Ctrl Pts',(28.,-0.449163693910779,5.65685424949238));
#60664=CARTESIAN_POINT('Ctrl Pts',(27.9882660485567,-0.936189504250083,
5.59576473572533));
#60665=CARTESIAN_POINT('Ctrl Pts',(27.941279648099,-1.8719981970442,5.3379209922756));
#60666=CARTESIAN_POINT('Ctrl Pts',(27.9063339848615,-2.32081120340133,5.14122028307955));
#60667=CARTESIAN_POINT('Ctrl Pts',(27.8289999774276,-3.11731851015347,4.66899487999358));
#60668=CARTESIAN_POINT('Ctrl Pts',(27.7822164601379,-3.50234534588973,4.36544996647722));
#60669=CARTESIAN_POINT('Ctrl Pts',(27.6879434354058,-4.18279363546962,3.6607064900872));
#60670=CARTESIAN_POINT('Ctrl Pts',(27.6406175296061,-4.47827306347342,3.25954202901027));
#60671=CARTESIAN_POINT('Ctrl Pts',(27.5182070810682,-5.19450970852415,1.96027825599731));
#60672=CARTESIAN_POINT('Ctrl Pts',(27.4666666666667,-5.4389541478323,0.960060375520684));
#60673=CARTESIAN_POINT('Ctrl Pts',(27.4666666666667,-5.4389541478323,-2.77555756156289E-16));
#60674=CARTESIAN_POINT('Origin',(0.,0.,0.));
#60675=CARTESIAN_POINT('',(18.4436057953749,-21.0673540166964,0.));
#60676=CARTESIAN_POINT('Origin',(0.,0.,0.));
#60677=CARTESIAN_POINT('',(10.4403065089456,-25.9807621135261,3.89989682781947));
#60678=CARTESIAN_POINT('Ctrl Pts',(18.4436057953749,-21.0673540166964,-2.77555756156289E-16));
#60679=CARTESIAN_POINT('Ctrl Pts',(18.4436057953749,-21.0673540166964,0.960060375520682));
#60680=CARTESIAN_POINT('Ctrl Pts',(18.2576809083209,-21.2342115445438,1.96027825599731));
#60681=CARTESIAN_POINT('Ctrl Pts',(17.6986070028546,-21.6983404251917,3.25954202901027));
#60682=CARTESIAN_POINT('Ctrl Pts',(17.4663772648075,-21.8870655758732,3.6607064900872));
#60683=CARTESIAN_POINT('Ctrl Pts',(16.9242282724357,-22.3089325549727,4.36544996647722));
#60684=CARTESIAN_POINT('Ctrl Pts',(16.6141770101942,-22.5419616872921,4.66899487999358));
#60685=CARTESIAN_POINT('Ctrl Pts',(15.9630484519639,-23.0071885556824,5.14122028307955));
#60686=CARTESIAN_POINT('Ctrl Pts',(15.5918378185284,-23.2618588909767,5.3379209922756));
#60687=CARTESIAN_POINT('Ctrl Pts',(14.8048969177153,-23.7704546538026,5.59576473572533));
#60688=CARTESIAN_POINT('Ctrl Pts',(14.3889871693844,-24.0241294590089,5.65685424949238));
#60689=CARTESIAN_POINT('Ctrl Pts',(13.6110128306156,-24.4732931529197,5.65685424949238));
#60690=CARTESIAN_POINT('Ctrl Pts',(13.1833691308414,-24.7066441580527,5.59576473572533));
#60691=CARTESIAN_POINT('Ctrl Pts',(12.3494418295706,-25.133857088021,5.3379209922756));
#60692=CARTESIAN_POINT('Ctrl Pts',(11.9432855328977,-25.3279997590838,5.14122028307955));
#60693=CARTESIAN_POINT('Ctrl Pts',(11.2148229672334,-25.6592801974456,4.66899487999358));
#60694=CARTESIAN_POINT('Ctrl Pts',(10.8579881877023,-25.8112779008625,4.36544996647722));
#60695=CARTESIAN_POINT('Ctrl Pts',(10.5061885578498,-25.9542157736402,3.97588378637689));
#60696=CARTESIAN_POINT('Ctrl Pts',(10.4730252750948,-25.9676141563614,3.93815105649065));
#60697=CARTESIAN_POINT('Ctrl Pts',(10.4403065089456,-25.9807621135191,3.89989682781947));
#60698=CARTESIAN_POINT('',(9.0230608712918,-26.5063081645287,0.));
#60699=CARTESIAN_POINT('Ctrl Pts',(10.4403065089456,-25.9807621135191,3.89989682781947));
#60700=CARTESIAN_POINT('Ctrl Pts',(10.1630550776949,-26.0921749315747,3.57573913794424));
#60701=CARTESIAN_POINT('Ctrl Pts',(9.9180326009165,-26.1854838629323,3.21382762602157));
#60702=CARTESIAN_POINT('Ctrl Pts',(9.2605261727473,-26.428721253068,1.96027825599731));
#60703=CARTESIAN_POINT('Ctrl Pts',(9.02306087129182,-26.5063081645287,0.960060375520684));
#60704=CARTESIAN_POINT('Ctrl Pts',(9.02306087129182,-26.5063081645287,-5.55111512312578E-16));
#60705=CARTESIAN_POINT('',(5.43895414783231,-27.4666666666667,0.));
#60706=CARTESIAN_POINT('Origin',(0.,0.,0.));
#60707=CARTESIAN_POINT('',(-5.43895414783233,-27.4666666666667,0.));
#60708=CARTESIAN_POINT('Ctrl Pts',(5.4389541478323,-27.4666666666667,0.));
#60709=CARTESIAN_POINT('Ctrl Pts',(5.4389541478323,-27.4666666666667,0.960060375520685));
#60710=CARTESIAN_POINT('Ctrl Pts',(5.19450970852414,-27.5182070810682,1.96027825599731));
#60711=CARTESIAN_POINT('Ctrl Pts',(4.47827306347341,-27.6406175296061,3.25954202901027));
#60712=CARTESIAN_POINT('Ctrl Pts',(4.18279363546962,-27.6879434354058,3.6607064900872));
#60713=CARTESIAN_POINT('Ctrl Pts',(3.50234534588972,-27.7822164601379,4.36544996647722));
#60714=CARTESIAN_POINT('Ctrl Pts',(3.11731851015346,-27.8289999774276,4.66899487999358));
#60715=CARTESIAN_POINT('Ctrl Pts',(2.32081120340132,-27.9063339848615,5.14122028307955));
#60716=CARTESIAN_POINT('Ctrl Pts',(1.87199819704419,-27.941279648099,5.3379209922756));
#60717=CARTESIAN_POINT('Ctrl Pts',(0.936189504250074,-27.9882660485567,
5.59576473572533));
#60718=CARTESIAN_POINT('Ctrl Pts',(0.449163693910773,-28.,5.65685424949238));
#60719=CARTESIAN_POINT('Ctrl Pts',(-0.449163693910784,-28.,5.65685424949238));
#60720=CARTESIAN_POINT('Ctrl Pts',(-0.936189504250087,-27.9882660485567,
5.59576473572533));
#60721=CARTESIAN_POINT('Ctrl Pts',(-1.87199819704421,-27.941279648099,5.3379209922756));
#60722=CARTESIAN_POINT('Ctrl Pts',(-2.32081120340134,-27.9063339848615,
5.14122028307955));
#60723=CARTESIAN_POINT('Ctrl Pts',(-3.11731851015348,-27.8289999774276,
4.66899487999358));
#60724=CARTESIAN_POINT('Ctrl Pts',(-3.50234534588974,-27.7822164601379,
4.36544996647722));
#60725=CARTESIAN_POINT('Ctrl Pts',(-4.18279363546963,-27.6879434354058,
3.6607064900872));
#60726=CARTESIAN_POINT('Ctrl Pts',(-4.47827306347343,-27.6406175296061,
3.25954202901027));
#60727=CARTESIAN_POINT('Ctrl Pts',(-5.19450970852415,-27.5182070810682,
1.96027825599731));
#60728=CARTESIAN_POINT('Ctrl Pts',(-5.43895414783231,-27.4666666666667,
0.960060375520684));
#60729=CARTESIAN_POINT('Ctrl Pts',(-5.43895414783231,-27.4666666666667,
-2.77555756156289E-16));
#60730=CARTESIAN_POINT('',(-9.02306087129181,-26.5063081645287,0.));
#60731=CARTESIAN_POINT('Origin',(0.,0.,0.));
#60732=CARTESIAN_POINT('',(-18.4436057953749,-21.0673540166964,0.));
#60733=CARTESIAN_POINT('Ctrl Pts',(-9.02306087129183,-26.5063081645287,
-2.77555756156289E-16));
#60734=CARTESIAN_POINT('Ctrl Pts',(-9.02306087129183,-26.5063081645287,
0.960060375520684));
#60735=CARTESIAN_POINT('Ctrl Pts',(-9.26052617274731,-26.428721253068,1.96027825599731));
#60736=CARTESIAN_POINT('Ctrl Pts',(-9.94201052675154,-26.1766134886651,
3.25954202901027));
#60737=CARTESIAN_POINT('Ctrl Pts',(-10.2215661705984,-26.0698592113429,
3.6607064900872));
#60738=CARTESIAN_POINT('Ctrl Pts',(-10.8579881877023,-25.8112779008625,
4.36544996647722));
#60739=CARTESIAN_POINT('Ctrl Pts',(-11.2148229672334,-25.6592801974456,
4.66899487999358));
#60740=CARTESIAN_POINT('Ctrl Pts',(-11.9432855328977,-25.3279997590838,
5.14122028307955));
#60741=CARTESIAN_POINT('Ctrl Pts',(-12.3494418295706,-25.1338570880209,
5.3379209922756));
#60742=CARTESIAN_POINT('Ctrl Pts',(-13.1833691308415,-24.7066441580527,
5.59576473572533));
#60743=CARTESIAN_POINT('Ctrl Pts',(-13.6110128306156,-24.4732931529197,
5.65685424949238));
#60744=CARTESIAN_POINT('Ctrl Pts',(-14.3889871693844,-24.0241294590089,
5.65685424949238));
#60745=CARTESIAN_POINT('Ctrl Pts',(-14.8048969177153,-23.7704546538026,
5.59576473572533));
#60746=CARTESIAN_POINT('Ctrl Pts',(-15.5918378185285,-23.2618588909767,
5.3379209922756));
#60747=CARTESIAN_POINT('Ctrl Pts',(-15.9630484519639,-23.0071885556824,
5.14122028307955));
#60748=CARTESIAN_POINT('Ctrl Pts',(-16.6141770101942,-22.5419616872921,
4.66899487999358));
#60749=CARTESIAN_POINT('Ctrl Pts',(-16.9242282724357,-22.3089325549727,
4.36544996647722));
#60750=CARTESIAN_POINT('Ctrl Pts',(-17.4663772648075,-21.8870655758732,
3.6607064900872));
#60751=CARTESIAN_POINT('Ctrl Pts',(-17.6986070028546,-21.6983404251917,
3.25954202901027));
#60752=CARTESIAN_POINT('Ctrl Pts',(-18.2576809083209,-21.2342115445438,
1.96027825599731));
#60753=CARTESIAN_POINT('Ctrl Pts',(-18.4436057953749,-21.0673540166964,
0.960060375520684));
#60754=CARTESIAN_POINT('Ctrl Pts',(-18.4436057953749,-21.0673540166964,
-5.55111512312578E-16));
#60755=CARTESIAN_POINT('',(-21.0673540166964,-18.4436057953749,0.));
#60756=CARTESIAN_POINT('Origin',(0.,0.,0.));
#60757=CARTESIAN_POINT('',(-26.5063081645287,-9.0230608712918,0.));
#60758=CARTESIAN_POINT('Ctrl Pts',(-21.0673540166964,-18.4436057953749,
-2.77555756156289E-16));
#60759=CARTESIAN_POINT('Ctrl Pts',(-21.0673540166964,-18.4436057953749,
0.960060375520684));
#60760=CARTESIAN_POINT('Ctrl Pts',(-21.2342115445438,-18.2576809083209,
1.96027825599731));
#60761=CARTESIAN_POINT('Ctrl Pts',(-21.6983404251917,-17.6986070028546,
3.25954202901027));
#60762=CARTESIAN_POINT('Ctrl Pts',(-21.8870655758732,-17.4663772648075,
3.6607064900872));
#60763=CARTESIAN_POINT('Ctrl Pts',(-22.3089325549727,-16.9242282724357,
4.36544996647722));
#60764=CARTESIAN_POINT('Ctrl Pts',(-22.5419616872921,-16.6141770101942,
4.66899487999358));
#60765=CARTESIAN_POINT('Ctrl Pts',(-23.0071885556824,-15.9630484519638,
5.14122028307955));
#60766=CARTESIAN_POINT('Ctrl Pts',(-23.2618588909767,-15.5918378185284,
5.3379209922756));
#60767=CARTESIAN_POINT('Ctrl Pts',(-23.7704546538026,-14.8048969177153,
5.59576473572534));
#60768=CARTESIAN_POINT('Ctrl Pts',(-24.0241294590089,-14.3889871693844,
5.65685424949239));
#60769=CARTESIAN_POINT('Ctrl Pts',(-24.4732931529197,-13.6110128306156,
5.65685424949239));
#60770=CARTESIAN_POINT('Ctrl Pts',(-24.7066441580527,-13.1833691308414,
5.59576473572533));
#60771=CARTESIAN_POINT('Ctrl Pts',(-25.1338570880209,-12.3494418295705,
5.33792099227561));
#60772=CARTESIAN_POINT('Ctrl Pts',(-25.3279997590838,-11.9432855328977,
5.14122028307956));
#60773=CARTESIAN_POINT('Ctrl Pts',(-25.6592801974456,-11.2148229672334,
4.66899487999359));
#60774=CARTESIAN_POINT('Ctrl Pts',(-25.8112779008625,-10.8579881877022,
4.36544996647723));
#60775=CARTESIAN_POINT('Ctrl Pts',(-26.0698592113429,-10.2215661705984,
3.66070649008721));
#60776=CARTESIAN_POINT('Ctrl Pts',(-26.1766134886651,-9.94201052675152,
3.25954202901028));
#60777=CARTESIAN_POINT('Ctrl Pts',(-26.428721253068,-9.26052617274729,1.96027825599731));
#60778=CARTESIAN_POINT('Ctrl Pts',(-26.5063081645287,-9.0230608712918,0.960060375520686));
#60779=CARTESIAN_POINT('Ctrl Pts',(-26.5063081645287,-9.0230608712918,-2.77555756156289E-16));
#60780=CARTESIAN_POINT('',(-27.4666666666667,-5.43895414783232,0.));
#60781=CARTESIAN_POINT('Origin',(0.,0.,0.));
#60782=CARTESIAN_POINT('Ctrl Pts',(-27.4666666666667,-5.4389541478323,-2.77555756156289E-16));
#60783=CARTESIAN_POINT('Ctrl Pts',(-27.4666666666667,-5.4389541478323,0.960060375520681));
#60784=CARTESIAN_POINT('Ctrl Pts',(-27.5182070810682,-5.19450970852415,
1.9602782559973));
#60785=CARTESIAN_POINT('Ctrl Pts',(-27.6406175296061,-4.47827306347342,
3.25954202901026));
#60786=CARTESIAN_POINT('Ctrl Pts',(-27.6879434354058,-4.18279363546963,
3.66070649008719));
#60787=CARTESIAN_POINT('Ctrl Pts',(-27.7822164601379,-3.50234534588974,
4.36544996647721));
#60788=CARTESIAN_POINT('Ctrl Pts',(-27.8289999774276,-3.11731851015348,
4.66899487999357));
#60789=CARTESIAN_POINT('Ctrl Pts',(-27.9063339848615,-2.32081120340134,
5.14122028307955));
#60790=CARTESIAN_POINT('Ctrl Pts',(-27.941279648099,-1.87199819704421,5.3379209922756));
#60791=CARTESIAN_POINT('Ctrl Pts',(-27.9882660485567,-0.936189504250084,
5.59576473572533));
#60792=CARTESIAN_POINT('Ctrl Pts',(-28.,-0.449163693910778,5.65685424949238));
#60793=CARTESIAN_POINT('Ctrl Pts',(-28.,3.88578058618805E-15,5.65685424949238));
#60794=CARTESIAN_POINT('Origin',(0.,0.,0.));
#60795=CARTESIAN_POINT('',(20.771851634051,-24.3419428085142,0.));
#60796=CARTESIAN_POINT('Origin',(0.,0.,0.));
#60797=CARTESIAN_POINT('Origin',(15.,-25.9807621135332,0.));
#60798=CARTESIAN_POINT('Origin',(15.,-25.9807621135332,0.));
#60799=CARTESIAN_POINT('',(10.6948150326157,-30.1599226029865,0.));
#60800=CARTESIAN_POINT('Ctrl Pts',(10.6948150326157,-30.1599226029865,2.77555756156289E-16));
#60801=CARTESIAN_POINT('Ctrl Pts',(10.6948150326157,-30.1599226029865,0.650190448083164));
#60802=CARTESIAN_POINT('Ctrl Pts',(10.811636102503,-30.1192963151694,1.34576815070429));
#60803=CARTESIAN_POINT('Ctrl Pts',(11.2845860623018,-29.945310285088,2.63799288444814));
#60804=CARTESIAN_POINT('Ctrl Pts',(11.6401587249113,-29.8110127779048,3.23471700046071));
#60805=CARTESIAN_POINT('Ctrl Pts',(12.2267378431101,-29.5727220114149,3.93620747216806));
#60806=CARTESIAN_POINT('Ctrl Pts',(12.4429603313741,-29.4828111958893,4.15945687249389));
#60807=CARTESIAN_POINT('Ctrl Pts',(12.9054296448663,-29.2833280818651,4.56176656225472));
#60808=CARTESIAN_POINT('Ctrl Pts',(13.1515948772024,-29.1736430103094,4.74086471477473));
#60809=CARTESIAN_POINT('Ctrl Pts',(13.7691022238565,-28.8892863729454,5.12459397949763));
#60810=CARTESIAN_POINT('Ctrl Pts',(14.2110789657823,-28.6758520004508,5.32832509625205));
#60811=CARTESIAN_POINT('Ctrl Pts',(15.116207912957,-28.2092096970821,5.59441429610713));
#60812=CARTESIAN_POINT('Ctrl Pts',(15.5792095317074,-27.9557564112432,5.65685424949238));
#60813=CARTESIAN_POINT('Ctrl Pts',(16.4207904682926,-27.4698694309609,5.65685424949238));
#60814=CARTESIAN_POINT('Ctrl Pts',(16.8717882618769,-27.1956249100491,5.59441429610713));
#60815=CARTESIAN_POINT('Ctrl Pts',(17.7284768246621,-26.6450813997796,5.32832509625205));
#60816=CARTESIAN_POINT('Ctrl Pts',(18.1343047842461,-26.3690354996372,5.12459397949762));
#60817=CARTESIAN_POINT('Ctrl Pts',(18.6893185292651,-25.9764367690933,4.74086471477472));
#60818=CARTESIAN_POINT('Ctrl Pts',(18.9073912038163,-25.8180939601396,4.56176656225471));
#60819=CARTESIAN_POINT('Ctrl Pts',(19.3113833049334,-25.5173253431967,4.15945687249388));
#60820=CARTESIAN_POINT('Ctrl Pts',(19.4973595993855,-25.3750265832533,3.93620747216806));
#60821=CARTESIAN_POINT('Ctrl Pts',(19.9970150157524,-24.9861795488087,3.23471700046071));
#60822=CARTESIAN_POINT('Ctrl Pts',(20.2911063999427,-24.7453933436892,2.63799288444813));
#60823=CARTESIAN_POINT('Ctrl Pts',(20.6782577017963,-24.4227996788253,1.34576815070429));
#60824=CARTESIAN_POINT('Ctrl Pts',(20.771851634051,-24.3419428085141,0.650190448083162));
#60825=CARTESIAN_POINT('Ctrl Pts',(20.771851634051,-24.3419428085141,-1.38777878078145E-16));
#60826=CARTESIAN_POINT('Origin',(15.,-25.9807621135332,0.));
#60827=CARTESIAN_POINT('',(15.,-25.9807621135332,6.));
#60828=CARTESIAN_POINT('Origin',(15.,-25.9807621135332,0.));
#60829=CARTESIAN_POINT('Origin',(0.,0.,0.));
#60830=CARTESIAN_POINT('',(5.81797979447235,-31.4666666666667,0.));
#60831=CARTESIAN_POINT('Origin',(0.,0.,0.));
#60832=CARTESIAN_POINT('Origin',(-5.55111512312578E-15,-30.,0.));
#60833=CARTESIAN_POINT('Origin',(-5.55111512312578E-15,-30.,0.));
#60834=CARTESIAN_POINT('',(-5.81797979447236,-31.4666666666667,0.));
#60835=CARTESIAN_POINT('Ctrl Pts',(-5.81797979447239,-31.4666666666667,
2.77555756156289E-16));
#60836=CARTESIAN_POINT('Ctrl Pts',(-5.81797979447239,-31.4666666666667,
0.650190448083165));
#60837=CARTESIAN_POINT('Ctrl Pts',(-5.69649663634415,-31.4898938042992,
1.34576815070429));
#60838=CARTESIAN_POINT('Ctrl Pts',(-5.1999169413988,-31.5756924622445,2.63799288444814));
#60839=CARTESIAN_POINT('Ctrl Pts',(-4.82483322909613,-31.6371737406638,
3.23471700046071));
#60840=CARTESIAN_POINT('Ctrl Pts',(-4.19769542816151,-31.7240974424956,
3.93620747216806));
#60841=CARTESIAN_POINT('Ctrl Pts',(-3.96548585269262,-31.7543436363075,
4.15945687249389));
#60842=CARTESIAN_POINT('Ctrl Pts',(-3.46523412172557,-31.8128208486826,
4.56176656225472));
#60843=CARTESIAN_POINT('Ctrl Pts',(-3.19720624121618,-31.8409134064675,
4.74086471477473));
#60844=CARTESIAN_POINT('Ctrl Pts',(-2.52025087330818,-31.9034070081026,
5.12459397949763));
#60845=CARTESIAN_POINT('Ctrl Pts',(-2.03077060067128,-31.9395557904444,
5.32832509625205));
#60846=CARTESIAN_POINT('Ctrl Pts',(-1.01358478703292,-31.9879961748339,
5.59441429610713));
#60847=CARTESIAN_POINT('Ctrl Pts',(-0.485886980282349,-32.,5.65685424949238));
#60848=CARTESIAN_POINT('Ctrl Pts',(0.485886980282342,-32.,5.65685424949238));
#60849=CARTESIAN_POINT('Ctrl Pts',(1.01358478703292,-31.9879961748339,5.59441429610713));
#60850=CARTESIAN_POINT('Ctrl Pts',(2.03077060067128,-31.9395557904444,5.32832509625205));
#60851=CARTESIAN_POINT('Ctrl Pts',(2.52025087330817,-31.9034070081026,5.12459397949762));
#60852=CARTESIAN_POINT('Ctrl Pts',(3.19720624121618,-31.8409134064675,4.74086471477472));
#60853=CARTESIAN_POINT('Ctrl Pts',(3.46523412172556,-31.8128208486826,4.56176656225471));
#60854=CARTESIAN_POINT('Ctrl Pts',(3.96548585269262,-31.7543436363075,4.15945687249388));
#60855=CARTESIAN_POINT('Ctrl Pts',(4.19769542816151,-31.7240974424956,3.93620747216805));
#60856=CARTESIAN_POINT('Ctrl Pts',(4.82483322909612,-31.6371737406638,3.2347170004607));
#60857=CARTESIAN_POINT('Ctrl Pts',(5.1999169413988,-31.5756924622445,2.63799288444813));
#60858=CARTESIAN_POINT('Ctrl Pts',(5.69649663634414,-31.4898938042993,1.34576815070429));
#60859=CARTESIAN_POINT('Ctrl Pts',(5.81797979447237,-31.4666666666667,0.650190448083162));
#60860=CARTESIAN_POINT('Ctrl Pts',(5.81797979447237,-31.4666666666667,-1.38777878078145E-16));
#60861=CARTESIAN_POINT('',(-6.00000000000001,-30.,0.));
#60862=CARTESIAN_POINT('Origin',(-5.55111512312578E-15,-30.,0.));
#60863=CARTESIAN_POINT('',(-5.91850916286999E-15,-30.,6.));
#60864=CARTESIAN_POINT('Origin',(-5.55111512312578E-15,-30.,0.));
#60865=CARTESIAN_POINT('Origin',(-5.55111512312578E-15,-30.,0.));
#60866=CARTESIAN_POINT('Origin',(0.,0.,0.));
#60867=CARTESIAN_POINT('',(-10.6948150326157,-30.1599226029865,0.));
#60868=CARTESIAN_POINT('Origin',(0.,0.,0.));
#60869=CARTESIAN_POINT('Origin',(-15.,-25.9807621135332,0.));
#60870=CARTESIAN_POINT('Origin',(-15.,-25.9807621135332,0.));
#60871=CARTESIAN_POINT('',(-20.771851634051,-24.3419428085142,0.));
#60872=CARTESIAN_POINT('',(-18.6815416923826,-25.9807621134925,4.73774743599203));
#60873=CARTESIAN_POINT('Ctrl Pts',(-20.771851634051,-24.3419428085141,-1.38777878078145E-16));
#60874=CARTESIAN_POINT('Ctrl Pts',(-20.771851634051,-24.3419428085141,0.650190448083165));
#60875=CARTESIAN_POINT('Ctrl Pts',(-20.6782577017963,-24.4227996788253,
1.3457681507043));
#60876=CARTESIAN_POINT('Ctrl Pts',(-20.2911063999427,-24.7453933436892,
2.63799288444815));
#60877=CARTESIAN_POINT('Ctrl Pts',(-19.9970150157524,-24.9861795488087,
3.23471700046072));
#60878=CARTESIAN_POINT('Ctrl Pts',(-19.4973595993855,-25.3750265832533,
3.93620747216807));
#60879=CARTESIAN_POINT('Ctrl Pts',(-19.3113833049334,-25.5173253431967,
4.1594568724939));
#60880=CARTESIAN_POINT('Ctrl Pts',(-18.9716143273131,-25.7702804014673,
4.49781089377006));
#60881=CARTESIAN_POINT('Ctrl Pts',(-18.8265576304416,-25.8764879862695,
4.6250605042284));
#60882=CARTESIAN_POINT('Ctrl Pts',(-18.6815416923826,-25.9807621134518,
4.73774743599203));
#60883=CARTESIAN_POINT('Origin',(-15.,-25.9807621135332,0.));
#60884=CARTESIAN_POINT('Ctrl Pts',(-18.6815416923826,-25.9807621134518,
4.73774743599203));
#60885=CARTESIAN_POINT('Ctrl Pts',(-18.6139422249284,-26.0293697048732,
4.79027667297257));
#60886=CARTESIAN_POINT('Ctrl Pts',(-18.5463811126206,-26.0775460638188,
4.83968978042875));
#60887=CARTESIAN_POINT('Ctrl Pts',(-18.1343047842461,-26.3690354996372,
5.12459397949763));
#60888=CARTESIAN_POINT('Ctrl Pts',(-17.7284768246621,-26.6450813997796,
5.32832509625205));
#60889=CARTESIAN_POINT('Ctrl Pts',(-16.8717882618769,-27.1956249100491,
5.59441429610713));
#60890=CARTESIAN_POINT('Ctrl Pts',(-16.4207904682926,-27.4698694309609,
5.65685424949238));
#60891=CARTESIAN_POINT('Ctrl Pts',(-15.5792095317074,-27.9557564112432,
5.65685424949238));
#60892=CARTESIAN_POINT('Ctrl Pts',(-15.116207912957,-28.2092096970821,5.59441429610713));
#60893=CARTESIAN_POINT('Ctrl Pts',(-14.2110789657823,-28.6758520004508,
5.32832509625205));
#60894=CARTESIAN_POINT('Ctrl Pts',(-13.7691022238565,-28.8892863729454,
5.12459397949763));
#60895=CARTESIAN_POINT('Ctrl Pts',(-13.1515948772024,-29.1736430103094,
4.74086471477473));
#60896=CARTESIAN_POINT('Ctrl Pts',(-12.9054296448663,-29.2833280818651,
4.56176656225472));
#60897=CARTESIAN_POINT('Ctrl Pts',(-12.4429603313742,-29.4828111958893,
4.15945687249389));
#60898=CARTESIAN_POINT('Ctrl Pts',(-12.2267378431101,-29.5727220114149,
3.93620747216806));
#60899=CARTESIAN_POINT('Ctrl Pts',(-11.6401587249113,-29.8110127779048,
3.23471700046071));
#60900=CARTESIAN_POINT('Ctrl Pts',(-11.2845860623018,-29.945310285088,2.63799288444814));
#60901=CARTESIAN_POINT('Ctrl Pts',(-10.811636102503,-30.1192963151694,1.3457681507043));
#60902=CARTESIAN_POINT('Ctrl Pts',(-10.6948150326157,-30.1599226029865,
0.650190448083164));
#60903=CARTESIAN_POINT('Ctrl Pts',(-10.6948150326157,-30.1599226029865,
-2.77555756156289E-16));
#60904=CARTESIAN_POINT('',(-15.,-25.9807621135332,6.));
#60905=CARTESIAN_POINT('Origin',(-15.,-25.9807621135332,0.));
#60906=CARTESIAN_POINT('Origin',(0.,0.,0.));
#60907=CARTESIAN_POINT('',(-24.3419428085141,-20.771851634051,0.));
#60908=CARTESIAN_POINT('Origin',(0.,0.,0.));
#60909=CARTESIAN_POINT('Origin',(-25.9807621135332,-15.,0.));
#60910=CARTESIAN_POINT('Origin',(-25.9807621135332,-15.,0.));
#60911=CARTESIAN_POINT('',(-30.1599226029865,-10.6948150326157,0.));
#60912=CARTESIAN_POINT('',(-28.2665880502059,-14.9999999999993,5.54752195013542));
#60913=CARTESIAN_POINT('Ctrl Pts',(-30.1599226029865,-10.6948150326157,
4.16333634234434E-16));
#60914=CARTESIAN_POINT('Ctrl Pts',(-30.1599226029865,-10.6948150326157,
0.650190448083161));
#60915=CARTESIAN_POINT('Ctrl Pts',(-30.1192963151694,-10.811636102503,1.34576815070429));
#60916=CARTESIAN_POINT('Ctrl Pts',(-29.945310285088,-11.2845860623018,2.63799288444813));
#60917=CARTESIAN_POINT('Ctrl Pts',(-29.8110127779048,-11.6401587249113,
3.2347170004607));
#60918=CARTESIAN_POINT('Ctrl Pts',(-29.5727220114149,-12.2267378431101,
3.93620747216805));
#60919=CARTESIAN_POINT('Ctrl Pts',(-29.4828111958893,-12.4429603313741,
4.15945687249388));
#60920=CARTESIAN_POINT('Ctrl Pts',(-29.2833280818651,-12.9054296448663,
4.56176656225471));
#60921=CARTESIAN_POINT('Ctrl Pts',(-29.1736430103094,-13.1515948772024,
4.74086471477472));
#60922=CARTESIAN_POINT('Ctrl Pts',(-28.8892863729454,-13.7691022238565,
5.12459397949763));
#60923=CARTESIAN_POINT('Ctrl Pts',(-28.6758520004509,-14.2110789657823,
5.32832509625205));
#60924=CARTESIAN_POINT('Ctrl Pts',(-28.3849162461088,-14.7753963693311,
5.49422274745779));
#60925=CARTESIAN_POINT('Ctrl Pts',(-28.3261413561496,-14.8877754155893,
5.52298333765861));
#60926=CARTESIAN_POINT('Ctrl Pts',(-28.2665880502059,-14.9999999999986,
5.54752195013542));
#60927=CARTESIAN_POINT('Origin',(-25.9807621135332,-15.,0.));
#60928=CARTESIAN_POINT('Ctrl Pts',(-28.2665880502059,-14.9999999999986,
5.54752195013542));
#60929=CARTESIAN_POINT('Ctrl Pts',(-28.0849690614805,-15.3422499424251,
5.62235705646812));
#60930=CARTESIAN_POINT('Ctrl Pts',(-27.8957657393658,-15.6831164233792,
5.65685424949238));
#60931=CARTESIAN_POINT('Ctrl Pts',(-27.4698694309609,-16.4207904682926,
5.65685424949238));
#60932=CARTESIAN_POINT('Ctrl Pts',(-27.1956249100492,-16.8717882618769,
5.59441429610713));
#60933=CARTESIAN_POINT('Ctrl Pts',(-26.6450813997796,-17.7284768246621,
5.32832509625206));
#60934=CARTESIAN_POINT('Ctrl Pts',(-26.3690354996372,-18.1343047842461,
5.12459397949763));
#60935=CARTESIAN_POINT('Ctrl Pts',(-25.9764367690933,-18.6893185292651,
4.74086471477474));
#60936=CARTESIAN_POINT('Ctrl Pts',(-25.8180939601396,-18.9073912038163,
4.56176656225472));
#60937=CARTESIAN_POINT('Ctrl Pts',(-25.5173253431967,-19.3113833049333,
4.1594568724939));
#60938=CARTESIAN_POINT('Ctrl Pts',(-25.3750265832534,-19.4973595993854,
3.93620747216807));
#60939=CARTESIAN_POINT('Ctrl Pts',(-24.9861795488087,-19.9970150157524,
3.23471700046072));
#60940=CARTESIAN_POINT('Ctrl Pts',(-24.7453933436892,-20.2911063999427,
2.63799288444814));
#60941=CARTESIAN_POINT('Ctrl Pts',(-24.4227996788253,-20.6782577017963,
1.3457681507043));
#60942=CARTESIAN_POINT('Ctrl Pts',(-24.3419428085142,-20.771851634051,0.650190448083165));
#60943=CARTESIAN_POINT('Ctrl Pts',(-24.3419428085142,-20.771851634051,0.));
#60944=CARTESIAN_POINT('',(-25.9807621135332,-15.,6.00000000000001));
#60945=CARTESIAN_POINT('Origin',(-25.9807621135332,-15.,0.));
#60946=CARTESIAN_POINT('Origin',(0.,0.,0.));
#60947=CARTESIAN_POINT('',(-31.4666666666667,-5.81797979447235,0.));
#60948=CARTESIAN_POINT('Origin',(0.,0.,0.));
#60949=CARTESIAN_POINT('Origin',(-30.,3.67394039744206E-15,0.));
#60950=CARTESIAN_POINT('Origin',(-30.,3.67394039744206E-15,0.));
#60951=CARTESIAN_POINT('',(-31.4666666666667,5.81797979447236,0.));
#60952=CARTESIAN_POINT('',(-32.,-2.97773713326802E-16,5.65685424949238));
#60953=CARTESIAN_POINT('Ctrl Pts',(-31.4666666666667,5.81797979447238,0.));
#60954=CARTESIAN_POINT('Ctrl Pts',(-31.4666666666667,5.81797979447238,0.650190448083164));
#60955=CARTESIAN_POINT('Ctrl Pts',(-31.4898938042993,5.69649663634415,1.34576815070429));
#60956=CARTESIAN_POINT('Ctrl Pts',(-31.5756924622445,5.1999169413988,2.63799288444814));
#60957=CARTESIAN_POINT('Ctrl Pts',(-31.6371737406638,4.82483322909612,3.23471700046071));
#60958=CARTESIAN_POINT('Ctrl Pts',(-31.7240974424956,4.19769542816151,3.93620747216806));
#60959=CARTESIAN_POINT('Ctrl Pts',(-31.7543436363075,3.96548585269262,4.15945687249389));
#60960=CARTESIAN_POINT('Ctrl Pts',(-31.8128208486826,3.46523412172556,4.56176656225472));
#60961=CARTESIAN_POINT('Ctrl Pts',(-31.8409134064675,3.19720624121618,4.74086471477473));
#60962=CARTESIAN_POINT('Ctrl Pts',(-31.9034070081026,2.52025087330817,5.12459397949763));
#60963=CARTESIAN_POINT('Ctrl Pts',(-31.9395557904444,2.03077060067128,5.32832509625205));
#60964=CARTESIAN_POINT('Ctrl Pts',(-31.9879961748339,1.01358478703292,5.59441429610713));
#60965=CARTESIAN_POINT('Ctrl Pts',(-32.,0.485886980282341,5.65685424949238));
#60966=CARTESIAN_POINT('Ctrl Pts',(-32.,-4.44089209850063E-15,5.65685424949238));
#60967=CARTESIAN_POINT('Origin',(-30.,3.67394039744206E-15,0.));
#60968=CARTESIAN_POINT('Ctrl Pts',(-32.,-3.88578058618805E-15,5.65685424949238));
#60969=CARTESIAN_POINT('Ctrl Pts',(-32.,-0.485886980282349,5.65685424949238));
#60970=CARTESIAN_POINT('Ctrl Pts',(-31.9879961748339,-1.01358478703293,
5.59441429610713));
#60971=CARTESIAN_POINT('Ctrl Pts',(-31.9395557904444,-2.03077060067129,
5.32832509625205));
#60972=CARTESIAN_POINT('Ctrl Pts',(-31.9034070081026,-2.52025087330818,
5.12459397949762));
#60973=CARTESIAN_POINT('Ctrl Pts',(-31.8409134064675,-3.19720624121619,
4.74086471477472));
#60974=CARTESIAN_POINT('Ctrl Pts',(-31.8128208486826,-3.46523412172557,
4.56176656225471));
#60975=CARTESIAN_POINT('Ctrl Pts',(-31.7543436363075,-3.96548585269263,
4.15945687249388));
#60976=CARTESIAN_POINT('Ctrl Pts',(-31.7240974424956,-4.19769542816152,
3.93620747216804));
#60977=CARTESIAN_POINT('Ctrl Pts',(-31.6371737406638,-4.82483322909613,
3.2347170004607));
#60978=CARTESIAN_POINT('Ctrl Pts',(-31.5756924622445,-5.1999169413988,2.63799288444813));
#60979=CARTESIAN_POINT('Ctrl Pts',(-31.4898938042993,-5.69649663634414,
1.34576815070429));
#60980=CARTESIAN_POINT('Ctrl Pts',(-31.4666666666667,-5.81797979447238,
0.65019044808316));
#60981=CARTESIAN_POINT('Ctrl Pts',(-31.4666666666667,-5.81797979447238,
-1.38777878078145E-16));
#60982=CARTESIAN_POINT('',(-30.,3.67394039744206E-15,6.));
#60983=CARTESIAN_POINT('Origin',(-30.,3.67394039744206E-15,0.));
#60984=CARTESIAN_POINT('Origin',(0.,0.,0.));
#60985=CARTESIAN_POINT('',(-30.1599226029865,10.6948150326157,0.));
#60986=CARTESIAN_POINT('Origin',(0.,0.,0.));
#60987=CARTESIAN_POINT('Origin',(-25.9807621135332,15.,0.));
#60988=CARTESIAN_POINT('Origin',(-25.9807621135332,15.,0.));
#60989=CARTESIAN_POINT('',(-24.3419428085142,20.771851634051,0.));
#60990=CARTESIAN_POINT('',(-28.2665880502059,14.9999999999993,5.54752195013541));
#60991=CARTESIAN_POINT('Ctrl Pts',(-24.3419428085142,20.771851634051,0.));
#60992=CARTESIAN_POINT('Ctrl Pts',(-24.3419428085142,20.771851634051,0.650190448083166));
#60993=CARTESIAN_POINT('Ctrl Pts',(-24.4227996788253,20.6782577017963,1.3457681507043));
#60994=CARTESIAN_POINT('Ctrl Pts',(-24.7453933436892,20.2911063999427,2.63799288444814));
#60995=CARTESIAN_POINT('Ctrl Pts',(-24.9861795488087,19.9970150157524,3.23471700046072));
#60996=CARTESIAN_POINT('Ctrl Pts',(-25.3750265832534,19.4973595993854,3.93620747216807));
#60997=CARTESIAN_POINT('Ctrl Pts',(-25.5173253431967,19.3113833049333,4.1594568724939));
#60998=CARTESIAN_POINT('Ctrl Pts',(-25.8180939601396,18.9073912038163,4.56176656225472));
#60999=CARTESIAN_POINT('Ctrl Pts',(-25.9764367690933,18.6893185292651,4.74086471477473));
#61000=CARTESIAN_POINT('Ctrl Pts',(-26.3690354996372,18.1343047842461,5.12459397949763));
#61001=CARTESIAN_POINT('Ctrl Pts',(-26.6450813997796,17.7284768246621,5.32832509625206));
#61002=CARTESIAN_POINT('Ctrl Pts',(-27.1956249100492,16.8717882618769,5.59441429610713));
#61003=CARTESIAN_POINT('Ctrl Pts',(-27.4698694309609,16.4207904682926,5.65685424949238));
#61004=CARTESIAN_POINT('Ctrl Pts',(-27.8957657393658,15.6831164233792,5.65685424949238));
#61005=CARTESIAN_POINT('Ctrl Pts',(-28.0849690614805,15.3422499424251,5.62235705646811));
#61006=CARTESIAN_POINT('Ctrl Pts',(-28.2665880502059,14.9999999999986,5.54752195013541));
#61007=CARTESIAN_POINT('Origin',(-25.9807621135332,15.,0.));
#61008=CARTESIAN_POINT('Ctrl Pts',(-28.2665880502059,14.9999999999986,5.54752195013541));
#61009=CARTESIAN_POINT('Ctrl Pts',(-28.3261413561496,14.8877754155893,5.52298333765861));
#61010=CARTESIAN_POINT('Ctrl Pts',(-28.3849162461088,14.7753963693311,5.49422274745778));
#61011=CARTESIAN_POINT('Ctrl Pts',(-28.6758520004509,14.2110789657823,5.32832509625205));
#61012=CARTESIAN_POINT('Ctrl Pts',(-28.8892863729454,13.7691022238565,5.12459397949762));
#61013=CARTESIAN_POINT('Ctrl Pts',(-29.1736430103094,13.1515948772024,4.74086471477472));
#61014=CARTESIAN_POINT('Ctrl Pts',(-29.2833280818651,12.9054296448663,4.56176656225471));
#61015=CARTESIAN_POINT('Ctrl Pts',(-29.4828111958893,12.4429603313741,4.15945687249387));
#61016=CARTESIAN_POINT('Ctrl Pts',(-29.5727220114149,12.2267378431101,3.93620747216804));
#61017=CARTESIAN_POINT('Ctrl Pts',(-29.8110127779048,11.6401587249113,3.23471700046069));
#61018=CARTESIAN_POINT('Ctrl Pts',(-29.945310285088,11.2845860623018,2.63799288444812));
#61019=CARTESIAN_POINT('Ctrl Pts',(-30.1192963151694,10.811636102503,1.34576815070429));
#61020=CARTESIAN_POINT('Ctrl Pts',(-30.1599226029865,10.6948150326157,0.650190448083159));
#61021=CARTESIAN_POINT('Ctrl Pts',(-30.1599226029865,10.6948150326157,-5.55111512312578E-16));
#61022=CARTESIAN_POINT('',(-25.9807621135332,15.,6.));
#61023=CARTESIAN_POINT('Origin',(-25.9807621135332,15.,0.));
#61024=CARTESIAN_POINT('Origin',(0.,0.,0.));
#61025=CARTESIAN_POINT('',(-20.771851634051,24.3419428085142,0.));
#61026=CARTESIAN_POINT('Origin',(0.,0.,0.));
#61027=CARTESIAN_POINT('Origin',(-15.,25.9807621135332,0.));
#61028=CARTESIAN_POINT('Origin',(-15.,25.9807621135332,0.));
#61029=CARTESIAN_POINT('',(-10.6948150326157,30.1599226029865,0.));
#61030=CARTESIAN_POINT('',(-18.6815416923826,25.9807621134925,4.73774743599202));
#61031=CARTESIAN_POINT('Ctrl Pts',(-10.6948150326157,30.1599226029865,-1.38777878078145E-16));
#61032=CARTESIAN_POINT('Ctrl Pts',(-10.6948150326157,30.1599226029865,0.650190448083162));
#61033=CARTESIAN_POINT('Ctrl Pts',(-10.811636102503,30.1192963151694,1.34576815070429));
#61034=CARTESIAN_POINT('Ctrl Pts',(-11.2845860623018,29.945310285088,2.63799288444813));
#61035=CARTESIAN_POINT('Ctrl Pts',(-11.6401587249113,29.8110127779048,3.2347170004607));
#61036=CARTESIAN_POINT('Ctrl Pts',(-12.2267378431101,29.5727220114149,3.93620747216805));
#61037=CARTESIAN_POINT('Ctrl Pts',(-12.4429603313741,29.4828111958893,4.15945687249388));
#61038=CARTESIAN_POINT('Ctrl Pts',(-12.9054296448663,29.2833280818651,4.56176656225471));
#61039=CARTESIAN_POINT('Ctrl Pts',(-13.1515948772024,29.1736430103094,4.74086471477472));
#61040=CARTESIAN_POINT('Ctrl Pts',(-13.7691022238565,28.8892863729454,5.12459397949762));
#61041=CARTESIAN_POINT('Ctrl Pts',(-14.2110789657823,28.6758520004509,5.32832509625205));
#61042=CARTESIAN_POINT('Ctrl Pts',(-15.116207912957,28.2092096970821,5.59441429610713));
#61043=CARTESIAN_POINT('Ctrl Pts',(-15.5792095317074,27.9557564112432,5.65685424949238));
#61044=CARTESIAN_POINT('Ctrl Pts',(-16.4207904682926,27.4698694309609,5.65685424949238));
#61045=CARTESIAN_POINT('Ctrl Pts',(-16.8717882618769,27.1956249100492,5.59441429610713));
#61046=CARTESIAN_POINT('Ctrl Pts',(-17.7284768246621,26.6450813997796,5.32832509625206));
#61047=CARTESIAN_POINT('Ctrl Pts',(-18.1343047842461,26.3690354996372,5.12459397949763));
#61048=CARTESIAN_POINT('Ctrl Pts',(-18.5463811126206,26.0775460638188,4.83968978042875));
#61049=CARTESIAN_POINT('Ctrl Pts',(-18.6139422249284,26.0293697048732,4.79027667297257));
#61050=CARTESIAN_POINT('Ctrl Pts',(-18.6815416923826,25.9807621134518,4.73774743599202));
#61051=CARTESIAN_POINT('Origin',(-15.,25.9807621135332,0.));
#61052=CARTESIAN_POINT('Ctrl Pts',(-18.6815416923826,25.9807621134518,4.73774743599202));
#61053=CARTESIAN_POINT('Ctrl Pts',(-18.8265576304416,25.8764879862695,4.6250605042284));
#61054=CARTESIAN_POINT('Ctrl Pts',(-18.9716143273131,25.7702804014673,4.49781089377006));
#61055=CARTESIAN_POINT('Ctrl Pts',(-19.3113833049333,25.5173253431967,4.1594568724939));
#61056=CARTESIAN_POINT('Ctrl Pts',(-19.4973595993854,25.3750265832534,3.93620747216807));
#61057=CARTESIAN_POINT('Ctrl Pts',(-19.9970150157524,24.9861795488087,3.23471700046072));
#61058=CARTESIAN_POINT('Ctrl Pts',(-20.2911063999427,24.7453933436892,2.63799288444815));
#61059=CARTESIAN_POINT('Ctrl Pts',(-20.6782577017962,24.4227996788253,1.3457681507043));
#61060=CARTESIAN_POINT('Ctrl Pts',(-20.771851634051,24.3419428085142,0.650190448083167));
#61061=CARTESIAN_POINT('Ctrl Pts',(-20.771851634051,24.3419428085142,-4.16333634234434E-16));
#61062=CARTESIAN_POINT('',(-15.,25.9807621135332,6.));
#61063=CARTESIAN_POINT('Origin',(-15.,25.9807621135332,0.));
#61064=CARTESIAN_POINT('Origin',(0.,0.,0.));
#61065=CARTESIAN_POINT('',(-5.81797979447235,31.4666666666667,0.));
#61066=CARTESIAN_POINT('Origin',(0.,0.,0.));
#61067=CARTESIAN_POINT('',(-6.,30.,0.));
#61068=CARTESIAN_POINT('Origin',(1.66533453693773E-15,30.,0.));
#61069=CARTESIAN_POINT('Origin',(1.66533453693773E-15,30.,0.));
#61070=CARTESIAN_POINT('Origin',(1.66533453693773E-15,30.,5.55111512312578E-16));
#61071=CARTESIAN_POINT('',(5.81797979447236,31.4666666666667,0.));
#61072=CARTESIAN_POINT('Ctrl Pts',(5.81797979447238,31.4666666666667,5.55111512312578E-16));
#61073=CARTESIAN_POINT('Ctrl Pts',(5.81797979447238,31.4666666666667,0.650190448083162));
#61074=CARTESIAN_POINT('Ctrl Pts',(5.69649663634414,31.4898938042992,1.34576815070429));
#61075=CARTESIAN_POINT('Ctrl Pts',(5.1999169413988,31.5756924622445,2.63799288444813));
#61076=CARTESIAN_POINT('Ctrl Pts',(4.82483322909613,31.6371737406637,3.2347170004607));
#61077=CARTESIAN_POINT('Ctrl Pts',(4.19769542816151,31.7240974424956,3.93620747216805));
#61078=CARTESIAN_POINT('Ctrl Pts',(3.96548585269263,31.7543436363075,4.15945687249388));
#61079=CARTESIAN_POINT('Ctrl Pts',(3.46523412172557,31.8128208486826,4.56176656225471));
#61080=CARTESIAN_POINT('Ctrl Pts',(3.19720624121618,31.8409134064675,4.74086471477472));
#61081=CARTESIAN_POINT('Ctrl Pts',(2.52025087330818,31.9034070081026,5.12459397949762));
#61082=CARTESIAN_POINT('Ctrl Pts',(2.03077060067129,31.9395557904444,5.32832509625205));
#61083=CARTESIAN_POINT('Ctrl Pts',(1.01358478703293,31.9879961748339,5.59441429610713));
#61084=CARTESIAN_POINT('Ctrl Pts',(0.485886980282349,32.,5.65685424949238));
#61085=CARTESIAN_POINT('Ctrl Pts',(-0.485886980282345,32.,5.65685424949238));
#61086=CARTESIAN_POINT('Ctrl Pts',(-1.01358478703292,31.9879961748339,5.59441429610713));
#61087=CARTESIAN_POINT('Ctrl Pts',(-2.03077060067128,31.9395557904444,5.32832509625205));
#61088=CARTESIAN_POINT('Ctrl Pts',(-2.52025087330818,31.9034070081026,5.12459397949762));
#61089=CARTESIAN_POINT('Ctrl Pts',(-3.19720624121618,31.8409134064675,4.74086471477472));
#61090=CARTESIAN_POINT('Ctrl Pts',(-3.46523412172557,31.8128208486826,4.56176656225471));
#61091=CARTESIAN_POINT('Ctrl Pts',(-3.96548585269262,31.7543436363075,4.15945687249388));
#61092=CARTESIAN_POINT('Ctrl Pts',(-4.19769542816151,31.7240974424956,3.93620747216805));
#61093=CARTESIAN_POINT('Ctrl Pts',(-4.82483322909612,31.6371737406638,3.23471700046071));
#61094=CARTESIAN_POINT('Ctrl Pts',(-5.1999169413988,31.5756924622445,2.63799288444813));
#61095=CARTESIAN_POINT('Ctrl Pts',(-5.69649663634414,31.4898938042993,1.34576815070429));
#61096=CARTESIAN_POINT('Ctrl Pts',(-5.81797979447238,31.4666666666667,0.650190448083163));
#61097=CARTESIAN_POINT('Ctrl Pts',(-5.81797979447238,31.4666666666667,1.38777878078145E-16));
#61098=CARTESIAN_POINT('Origin',(1.66533453693773E-15,30.,0.));
#61099=CARTESIAN_POINT('',(1.29794049719353E-15,30.,6.));
#61100=CARTESIAN_POINT('Origin',(1.66533453693773E-15,30.,5.55111512312578E-16));
#61101=CARTESIAN_POINT('Origin',(0.,0.,0.));
#61102=CARTESIAN_POINT('',(10.6948150326157,30.1599226029865,0.));
#61103=CARTESIAN_POINT('Origin',(0.,0.,0.));
#61104=CARTESIAN_POINT('Origin',(15.,25.9807621135332,0.));
#61105=CARTESIAN_POINT('Origin',(15.,25.9807621135332,0.));
#61106=CARTESIAN_POINT('',(20.771851634051,24.3419428085142,0.));
#61107=CARTESIAN_POINT('Ctrl Pts',(20.771851634051,24.3419428085141,-5.55111512312578E-16));
#61108=CARTESIAN_POINT('Ctrl Pts',(20.771851634051,24.3419428085141,0.650190448083163));
#61109=CARTESIAN_POINT('Ctrl Pts',(20.6782577017963,24.4227996788253,1.34576815070429));
#61110=CARTESIAN_POINT('Ctrl Pts',(20.2911063999427,24.7453933436892,2.63799288444813));
#61111=CARTESIAN_POINT('Ctrl Pts',(19.9970150157524,24.9861795488087,3.23471700046071));
#61112=CARTESIAN_POINT('Ctrl Pts',(19.4973595993855,25.3750265832533,3.93620747216806));
#61113=CARTESIAN_POINT('Ctrl Pts',(19.3113833049334,25.5173253431967,4.15945687249388));
#61114=CARTESIAN_POINT('Ctrl Pts',(18.9073912038163,25.8180939601395,4.56176656225471));
#61115=CARTESIAN_POINT('Ctrl Pts',(18.6893185292651,25.9764367690933,4.74086471477473));
#61116=CARTESIAN_POINT('Ctrl Pts',(18.1343047842461,26.3690354996372,5.12459397949762));
#61117=CARTESIAN_POINT('Ctrl Pts',(17.7284768246621,26.6450813997796,5.32832509625205));
#61118=CARTESIAN_POINT('Ctrl Pts',(16.8717882618769,27.1956249100491,5.59441429610713));
#61119=CARTESIAN_POINT('Ctrl Pts',(16.4207904682926,27.4698694309609,5.65685424949238));
#61120=CARTESIAN_POINT('Ctrl Pts',(15.5792095317074,27.9557564112432,5.65685424949238));
#61121=CARTESIAN_POINT('Ctrl Pts',(15.116207912957,28.2092096970821,5.59441429610713));
#61122=CARTESIAN_POINT('Ctrl Pts',(14.2110789657823,28.6758520004508,5.32832509625205));
#61123=CARTESIAN_POINT('Ctrl Pts',(13.7691022238565,28.8892863729454,5.12459397949763));
#61124=CARTESIAN_POINT('Ctrl Pts',(13.1515948772024,29.1736430103094,4.74086471477473));
#61125=CARTESIAN_POINT('Ctrl Pts',(12.9054296448663,29.2833280818651,4.56176656225472));
#61126=CARTESIAN_POINT('Ctrl Pts',(12.4429603313741,29.4828111958893,4.15945687249389));
#61127=CARTESIAN_POINT('Ctrl Pts',(12.2267378431101,29.5727220114149,3.93620747216806));
#61128=CARTESIAN_POINT('Ctrl Pts',(11.6401587249113,29.8110127779048,3.23471700046071));
#61129=CARTESIAN_POINT('Ctrl Pts',(11.2845860623018,29.945310285088,2.63799288444813));
#61130=CARTESIAN_POINT('Ctrl Pts',(10.811636102503,30.1192963151694,1.34576815070429));
#61131=CARTESIAN_POINT('Ctrl Pts',(10.6948150326157,30.1599226029865,0.650190448083163));
#61132=CARTESIAN_POINT('Ctrl Pts',(10.6948150326157,30.1599226029865,1.38777878078145E-16));
#61133=CARTESIAN_POINT('Origin',(15.,25.9807621135332,0.));
#61134=CARTESIAN_POINT('',(15.,25.9807621135332,6.));
#61135=CARTESIAN_POINT('Origin',(15.,25.9807621135332,0.));
#61136=CARTESIAN_POINT('Origin',(0.,0.,0.));
#61137=CARTESIAN_POINT('',(24.3419428085142,20.771851634051,0.));
#61138=CARTESIAN_POINT('Origin',(0.,0.,0.));
#61139=CARTESIAN_POINT('Origin',(25.9807621135332,15.,0.));
#61140=CARTESIAN_POINT('Origin',(25.9807621135332,15.,0.));
#61141=CARTESIAN_POINT('',(30.1599226029865,10.6948150326157,0.));
#61142=CARTESIAN_POINT('Ctrl Pts',(30.1599226029865,10.6948150326157,-4.16333634234434E-16));
#61143=CARTESIAN_POINT('Ctrl Pts',(30.1599226029865,10.6948150326157,0.650190448083162));
#61144=CARTESIAN_POINT('Ctrl Pts',(30.1192963151694,10.811636102503,1.34576815070429));
#61145=CARTESIAN_POINT('Ctrl Pts',(29.945310285088,11.2845860623018,2.63799288444813));
#61146=CARTESIAN_POINT('Ctrl Pts',(29.8110127779048,11.6401587249113,3.23471700046071));
#61147=CARTESIAN_POINT('Ctrl Pts',(29.5727220114149,12.2267378431101,3.93620747216805));
#61148=CARTESIAN_POINT('Ctrl Pts',(29.4828111958893,12.4429603313741,4.15945687249388));
#61149=CARTESIAN_POINT('Ctrl Pts',(29.2833280818651,12.9054296448663,4.56176656225471));
#61150=CARTESIAN_POINT('Ctrl Pts',(29.1736430103094,13.1515948772024,4.74086471477472));
#61151=CARTESIAN_POINT('Ctrl Pts',(28.8892863729454,13.7691022238565,5.12459397949762));
#61152=CARTESIAN_POINT('Ctrl Pts',(28.6758520004509,14.2110789657823,5.32832509625205));
#61153=CARTESIAN_POINT('Ctrl Pts',(28.2092096970821,15.116207912957,5.59441429610713));
#61154=CARTESIAN_POINT('Ctrl Pts',(27.9557564112432,15.5792095317074,5.65685424949238));
#61155=CARTESIAN_POINT('Ctrl Pts',(27.4698694309609,16.4207904682926,5.65685424949238));
#61156=CARTESIAN_POINT('Ctrl Pts',(27.1956249100492,16.8717882618769,5.59441429610713));
#61157=CARTESIAN_POINT('Ctrl Pts',(26.6450813997796,17.7284768246621,5.32832509625205));
#61158=CARTESIAN_POINT('Ctrl Pts',(26.3690354996372,18.1343047842461,5.12459397949763));
#61159=CARTESIAN_POINT('Ctrl Pts',(25.9764367690933,18.6893185292651,4.74086471477473));
#61160=CARTESIAN_POINT('Ctrl Pts',(25.8180939601396,18.9073912038163,4.56176656225471));
#61161=CARTESIAN_POINT('Ctrl Pts',(25.5173253431967,19.3113833049334,4.15945687249389));
#61162=CARTESIAN_POINT('Ctrl Pts',(25.3750265832534,19.4973595993854,3.93620747216806));
#61163=CARTESIAN_POINT('Ctrl Pts',(24.9861795488087,19.9970150157524,3.23471700046071));
#61164=CARTESIAN_POINT('Ctrl Pts',(24.7453933436892,20.2911063999427,2.63799288444814));
#61165=CARTESIAN_POINT('Ctrl Pts',(24.4227996788253,20.6782577017963,1.34576815070429));
#61166=CARTESIAN_POINT('Ctrl Pts',(24.3419428085142,20.771851634051,0.650190448083164));
#61167=CARTESIAN_POINT('Ctrl Pts',(24.3419428085142,20.771851634051,-2.77555756156289E-16));
#61168=CARTESIAN_POINT('Origin',(25.9807621135332,15.,0.));
#61169=CARTESIAN_POINT('',(25.9807621135332,15.,6.));
#61170=CARTESIAN_POINT('Origin',(25.9807621135332,15.,0.));
#61171=CARTESIAN_POINT('Origin',(0.,0.,0.));
#61172=CARTESIAN_POINT('',(31.4666666666667,5.81797979447236,0.));
#61173=CARTESIAN_POINT('Origin',(0.,0.,0.));
#61174=CARTESIAN_POINT('Origin',(30.,0.,0.));
#61175=CARTESIAN_POINT('Origin',(30.,0.,0.));
#61176=CARTESIAN_POINT('',(31.4666666666667,-5.81797979447236,0.));
#61177=CARTESIAN_POINT('Ctrl Pts',(31.4666666666667,-5.81797979447238,1.38777878078145E-16));
#61178=CARTESIAN_POINT('Ctrl Pts',(31.4666666666667,-5.81797979447238,0.650190448083163));
#61179=CARTESIAN_POINT('Ctrl Pts',(31.4898938042993,-5.69649663634414,1.34576815070429));
#61180=CARTESIAN_POINT('Ctrl Pts',(31.5756924622445,-5.1999169413988,2.63799288444813));
#61181=CARTESIAN_POINT('Ctrl Pts',(31.6371737406638,-4.82483322909612,3.23471700046071));
#61182=CARTESIAN_POINT('Ctrl Pts',(31.7240974424956,-4.19769542816151,3.93620747216806));
#61183=CARTESIAN_POINT('Ctrl Pts',(31.7543436363075,-3.96548585269262,4.15945687249389));
#61184=CARTESIAN_POINT('Ctrl Pts',(31.8128208486826,-3.46523412172556,4.56176656225471));
#61185=CARTESIAN_POINT('Ctrl Pts',(31.8409134064675,-3.19720624121618,4.74086471477473));
#61186=CARTESIAN_POINT('Ctrl Pts',(31.9034070081026,-2.52025087330817,5.12459397949763));
#61187=CARTESIAN_POINT('Ctrl Pts',(31.9395557904444,-2.03077060067128,5.32832509625205));
#61188=CARTESIAN_POINT('Ctrl Pts',(31.9879961748339,-1.01358478703292,5.59441429610713));
#61189=CARTESIAN_POINT('Ctrl Pts',(32.,-0.485886980282346,5.65685424949238));
#61190=CARTESIAN_POINT('Ctrl Pts',(32.,0.485886980282346,5.65685424949238));
#61191=CARTESIAN_POINT('Ctrl Pts',(31.9879961748339,1.01358478703292,5.59441429610713));
#61192=CARTESIAN_POINT('Ctrl Pts',(31.9395557904444,2.03077060067128,5.32832509625205));
#61193=CARTESIAN_POINT('Ctrl Pts',(31.9034070081026,2.52025087330817,5.12459397949763));
#61194=CARTESIAN_POINT('Ctrl Pts',(31.8409134064675,3.19720624121618,4.74086471477473));
#61195=CARTESIAN_POINT('Ctrl Pts',(31.8128208486826,3.46523412172556,4.56176656225471));
#61196=CARTESIAN_POINT('Ctrl Pts',(31.7543436363075,3.96548585269262,4.15945687249389));
#61197=CARTESIAN_POINT('Ctrl Pts',(31.7240974424956,4.19769542816151,3.93620747216806));
#61198=CARTESIAN_POINT('Ctrl Pts',(31.6371737406638,4.82483322909612,3.23471700046071));
#61199=CARTESIAN_POINT('Ctrl Pts',(31.5756924622445,5.1999169413988,2.63799288444813));
#61200=CARTESIAN_POINT('Ctrl Pts',(31.4898938042993,5.69649663634414,1.34576815070429));
#61201=CARTESIAN_POINT('Ctrl Pts',(31.4666666666667,5.81797979447238,0.650190448083162));
#61202=CARTESIAN_POINT('Ctrl Pts',(31.4666666666667,5.81797979447238,-2.77555756156289E-16));
#61203=CARTESIAN_POINT('Origin',(30.,0.,0.));
#61204=CARTESIAN_POINT('',(30.,-4.49927934798557E-32,6.));
#61205=CARTESIAN_POINT('Origin',(30.,0.,0.));
#61206=CARTESIAN_POINT('Origin',(0.,0.,0.));
#61207=CARTESIAN_POINT('',(-32.,-3.91886975727153E-15,8.));
#61208=CARTESIAN_POINT('Origin',(0.,0.,8.));
#61209=CARTESIAN_POINT('',(-32.,-3.91886975727153E-15,0.));
#61210=CARTESIAN_POINT('Origin',(0.,0.,0.));
#61211=CARTESIAN_POINT('Origin',(0.,0.,8.));
#61212=CARTESIAN_POINT('Origin',(0.,0.,0.));
#63875=UNCERTAINTY_MEASURE_WITH_UNIT(LENGTH_MEASURE(0.01),#63899,
'DISTANCE_ACCURACY_VALUE',
'Maximum model space distance between geometric entities at asserted c
onnectivities');
#63878=UNCERTAINTY_MEASURE_WITH_UNIT(LENGTH_MEASURE(0.01),#63899,
'DISTANCE_ACCURACY_VALUE',
'Maximum model space distance between geometric entities at asserted c
onnectivities');
#63895=(
GEOMETRIC_REPRESENTATION_CONTEXT(3)
GLOBAL_UNCERTAINTY_ASSIGNED_CONTEXT((#63875))
GLOBAL_UNIT_ASSIGNED_CONTEXT((#63899,#63901,#63902))
REPRESENTATION_CONTEXT('','3D')
);
#63898=(
GEOMETRIC_REPRESENTATION_CONTEXT(3)
GLOBAL_UNCERTAINTY_ASSIGNED_CONTEXT((#63878))
GLOBAL_UNIT_ASSIGNED_CONTEXT((#63899,#63901,#63902))
REPRESENTATION_CONTEXT('','3D')
);
#63899=(
LENGTH_UNIT()
NAMED_UNIT(*)
SI_UNIT(.MILLI.,.METRE.)
);
#63901=(
NAMED_UNIT(*)
PLANE_ANGLE_UNIT()
SI_UNIT($,.RADIAN.)
);
#63902=(
NAMED_UNIT(*)
SI_UNIT($,.STERADIAN.)
SOLID_ANGLE_UNIT()
);
#63919=SHAPE_DEFINITION_REPRESENTATION(#63938,#64010);
#63938=PRODUCT_DEFINITION_SHAPE('',$,#64030);
#64010=SHAPE_REPRESENTATION('',(#16651),#63895);
#64013=PRODUCT_DEFINITION_CONTEXT('part definition',#64072,'design');
#64030=PRODUCT_DEFINITION('Ball cage','Ball cage',#64049,#64013);
#64049=PRODUCT_DEFINITION_FORMATION('',$,#64090);
#64072=APPLICATION_CONTEXT(
'Core Data for Automotive Mechanical Design Process');
#64073=PRODUCT_CONTEXT('part definition',#64072,'mechanical');
#64090=PRODUCT('Ball cage','Ball cage',$,(#64073));
#64105=PRESENTATION_STYLE_ASSIGNMENT((#64118));
#64118=SURFACE_STYLE_USAGE(.BOTH.,#64131);
#64131=SURFACE_SIDE_STYLE('',(#64144));
#64144=SURFACE_STYLE_FILL_AREA(#64157);
#64157=FILL_AREA_STYLE('Cage dark gray',(#64170));
#64170=FILL_AREA_STYLE_COLOUR('Cage dark gray',#64183);
#64183=COLOUR_RGB('Cage dark gray',0.250980392156863,0.282352941176471,
0.32156862745098);
ENDSEC;
END-ISO-10303-21;
